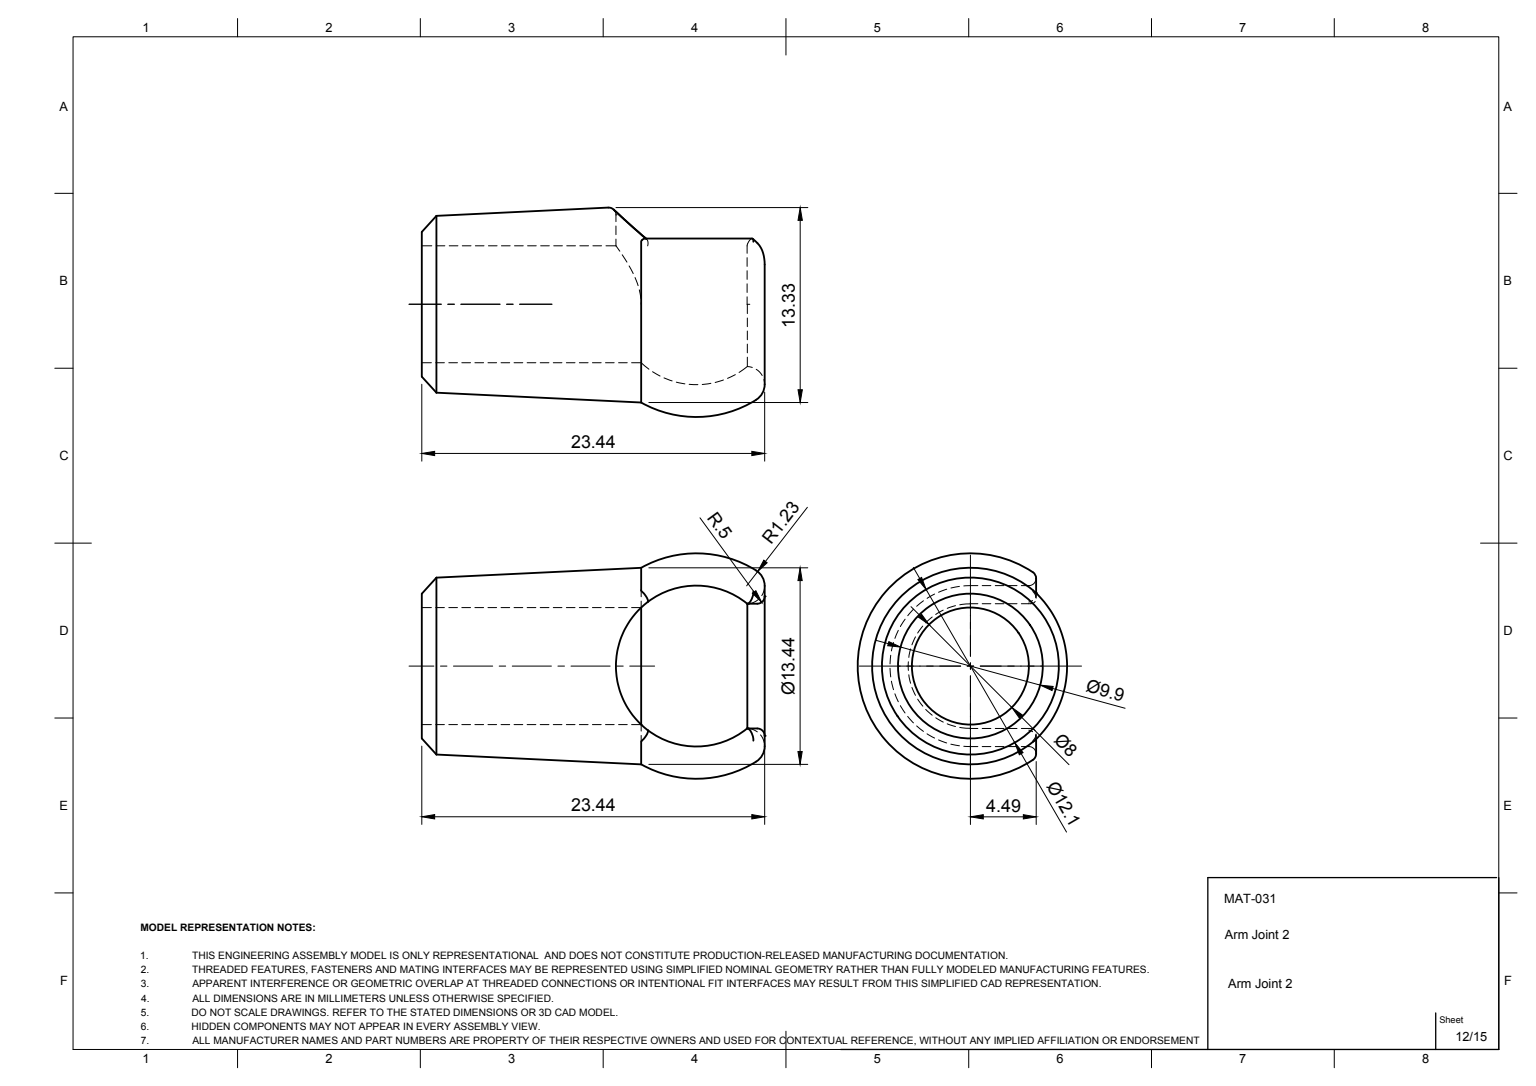
ISO-10303-21;
HEADER;
/* Generated by software containing ST-Developer
 * from STEP Tools, Inc. (www.steptools.com) 
 */

FILE_DESCRIPTION(
/* description */ ('STEP AP214'),
/* implementation_level */ '2;1');

FILE_NAME(
/* name */ 'Arm Joint 2.step',
/* time_stamp */ '2026-11-14T06:58:01-08:00',
/* author */ (''),
/* organization */ (''),
/* preprocessor_version */ 'ST-DEVELOPER v20.2',
/* originating_system */ 'Autodesk Translation Framework v15.17.0.0',
/* authorisation */ '');

FILE_SCHEMA (('AUTOMOTIVE_DESIGN { 1 0 10303 214 3 1 1 }'));
ENDSEC;

DATA;
#10=MECHANICAL_DESIGN_GEOMETRIC_PRESENTATION_REPRESENTATION('',(#1155),#38635);
#89=SPHERICAL_SURFACE('',#18166,5.5);
#90=SPHERICAL_SURFACE('',#18175,7.70789157434132);
#135=(
BOUNDED_SURFACE()
B_SPLINE_SURFACE(3,2,((#32683,#32684,#32685),(#32686,#32687,#32688),(#32689,
#32690,#32691),(#32692,#32693,#32694),(#32695,#32696,#32697),(#32698,#32699,
#32700),(#32701,#32702,#32703),(#32704,#32705,#32706),(#32707,#32708,#32709),
(#32710,#32711,#32712),(#32713,#32714,#32715),(#32716,#32717,#32718),(#32719,
#32720,#32721),(#32722,#32723,#32724),(#32725,#32726,#32727),(#32728,#32729,
#32730),(#32731,#32732,#32733),(#32734,#32735,#32736),(#32737,#32738,#32739),
(#32740,#32741,#32742),(#32743,#32744,#32745),(#32746,#32747,#32748)),
 .UNSPECIFIED.,.F.,.F.,.F.)
B_SPLINE_SURFACE_WITH_KNOTS((4,2,2,2,2,2,2,2,2,2,4),(3,3),(0.00881272913566369,
0.00928844068390005,0.00953838644963798,0.00978833221537591,0.0100382779811138,
0.0105381695125897,0.0110380610440656,0.0120378441070173,0.0125377356384932,
0.0127876814042311,0.01326339295247),(-0.00102566064560791,1.),
 .UNSPECIFIED.)
GEOMETRIC_REPRESENTATION_ITEM()
RATIONAL_B_SPLINE_SURFACE(((1.00132329066919,0.354908139032077,1.),(1.00124812393843,
0.391551219315617,1.),(1.00115915858371,0.434921000104149,1.),(1.00102358876472,
0.501010022609669,1.),(1.00097653790903,0.523946875988812,1.),(1.00088693501083,
0.567627453274935,1.),(1.00084389129738,0.588610862181495,1.),(1.00076096626522,
0.629036042047148,1.),(1.00072089412048,0.648570838919578,1.),(1.00060683104295,
0.704175525527758,1.),(1.00053863758583,0.737419199938388,1.),(1.00041471240488,
0.797831569997033,1.),(1.00035895931741,0.825010680216488,1.),(1.00021007792585,
0.897588970214807,1.),(1.00013587466058,0.933762370057051,1.),(1.00006032673641,
0.970591278572527,1.),(1.00004117816685,0.979926027666627,1.),(1.00002165568508,
0.989443055473061,1.),(1.00001667885161,0.991869215376876,1.),(1.00000682799133,
0.99667141789903,1.),(1.00000607453102,0.997038722775045,1.),(1.00001271218793,
0.993802926931325,1.)))
REPRESENTATION_ITEM('')
SURFACE()
);
#136=(
BOUNDED_SURFACE()
B_SPLINE_SURFACE(3,2,((#32822,#32823,#32824),(#32825,#32826,#32827),(#32828,
#32829,#32830),(#32831,#32832,#32833),(#32834,#32835,#32836),(#32837,#32838,
#32839),(#32840,#32841,#32842),(#32843,#32844,#32845),(#32846,#32847,#32848),
(#32849,#32850,#32851),(#32852,#32853,#32854),(#32855,#32856,#32857),(#32858,
#32859,#32860),(#32861,#32862,#32863),(#32864,#32865,#32866),(#32867,#32868,
#32869),(#32870,#32871,#32872),(#32873,#32874,#32875),(#32876,#32877,#32878),
(#32879,#32880,#32881),(#32882,#32883,#32884),(#32885,#32886,#32887),(#32888,
#32889,#32890),(#32891,#32892,#32893),(#32894,#32895,#32896),(#32897,#32898,
#32899),(#32900,#32901,#32902),(#32903,#32904,#32905)),.UNSPECIFIED.,.F.,
 .F.,.F.)
B_SPLINE_SURFACE_WITH_KNOTS((4,2,2,2,2,2,2,2,2,2,2,2,2,4),(3,3),(0.0120978781599544,
0.013608206651586,0.0151185351432177,0.0158736993890335,0.0166288636348494,
0.0173840278806652,0.018139192126481,0.0188943563722969,0.0196495206181127,
0.0204046848639285,0.0211598491097444,0.0219150133555602,0.022670177601376,
0.0241805060930077),(0.,1.00005676629322),.UNSPECIFIED.)
GEOMETRIC_REPRESENTATION_ITEM()
RATIONAL_B_SPLINE_SURFACE(((1.,0.419714375858336,1.00006588132778),(1.,
0.455258548961405,1.00006184590587),(1.,0.490259453324333,1.00005787216267),
(1.,0.554227398223351,1.00005060971644),(1.,0.583234396585999,1.00004731647689),
(1.,0.620852932125695,1.00004304554726),(1.,0.632335513594305,1.00004174190008),
(1.,0.652343207191375,1.00003947037488),(1.,0.660962788243787,1.00003849177155),
(1.,0.67512712292899,1.000036883658),(1.,0.680682058163542,1.00003625299183),
(1.,0.688032273240624,1.0000354185029),(1.,0.689900381447712,1.00003520641175),
(1.,0.689947597716664,1.00003520105116),(1.,0.688072411855674,1.00003541394586),
(1.,0.680752669873931,1.0000362449751),(1.,0.675339625853613,1.00003685953199),
(1.,0.661242565913974,1.00003846000767),(1.,0.652474855221301,1.00003945542854),
(1.,0.632370855573539,1.00004173788762),(1.,0.621020695612542,1.00004302650063),
(1.,0.596023875522447,1.00004586445427),(1.,0.582284387510476,1.00004742433388),
(1.,0.553320360279571,1.00005071269481),(1.,0.538073094759082,1.0000524437563),
(1.,0.490378194191559,1.00005785868172),(1.,0.455940368475232,1.00006176849714),
(1.,0.419656970284633,1.00006588784518)))
REPRESENTATION_ITEM('')
SURFACE()
);
#137=(
BOUNDED_SURFACE()
B_SPLINE_SURFACE(3,2,((#32908,#32909,#32910),(#32911,#32912,#32913),(#32914,
#32915,#32916),(#32917,#32918,#32919),(#32920,#32921,#32922),(#32923,#32924,
#32925),(#32926,#32927,#32928),(#32929,#32930,#32931),(#32932,#32933,#32934),
(#32935,#32936,#32937),(#32938,#32939,#32940),(#32941,#32942,#32943),(#32944,
#32945,#32946),(#32947,#32948,#32949),(#32950,#32951,#32952),(#32953,#32954,
#32955),(#32956,#32957,#32958),(#32959,#32960,#32961),(#32962,#32963,#32964),
(#32965,#32966,#32967),(#32968,#32969,#32970),(#32971,#32972,#32973)),
 .UNSPECIFIED.,.F.,.F.,.F.)
B_SPLINE_SURFACE_WITH_KNOTS((4,2,2,2,2,2,2,2,2,2,4),(3,3),(0.0086385816929815,
0.00928844068390017,0.00953838644963812,0.00978833221537607,0.010038277981114,
0.0105381695125899,0.0110380610440658,0.0120378441070176,0.0125377356384935,
0.0127876814042315,0.0134375403951501),(0.,1.00153795011474),
 .UNSPECIFIED.)
GEOMETRIC_REPRESENTATION_ITEM()
RATIONAL_B_SPLINE_SURFACE(((1.,0.317352891590616,1.0020997543974),(1.,0.359464191769642,
1.00197022423952),(1.,0.418763269709159,1.00178782619208),(1.,0.50075465721736,
1.00153562886443),(1.,0.523703248865329,1.00146504128611),(1.,0.567406180323521,
1.00133061542921),(1.,0.588400327795338,1.00126603952618),(1.,0.628846195835825,
1.0011416320714),(1.,0.648390989925248,1.00108151423477),(1.,0.704024133042094,
1.00091039223709),(1.,0.737284820387534,1.00080808568126),(1.,0.797728107356911,
1.000622168161),(1.,0.82492112688211,1.000538525146),(1.,0.897536559877894,
1.00031516731898),(1.,0.933728471984707,1.00020384460823),(1.,0.970576228230773,
1.00009050458634),(1.,0.97991575451876,1.00006177713528),(1.,0.98943765280286,
1.00003248872617),(1.,0.991865054329365,1.00002502228126),(1.,0.997822764595849,
1.00000669695888),(1.,0.996933411986155,1.00000943251877),(1.,0.988754588874827,
1.00003458976266)))
REPRESENTATION_ITEM('')
SURFACE()
);
#149=TOROIDAL_SURFACE('',#18150,6.,0.5);
#150=TOROIDAL_SURFACE('',#18161,5.48772230081581,1.23243402184158);
#151=TOROIDAL_SURFACE('',#18192,5.40661052483917,0.5);
#152=TOROIDAL_SURFACE('',#18193,6.,0.5);
#153=TOROIDAL_SURFACE('',#18194,5.40661052483917,0.5);
#878=FACE_BOUND('',#2883,.T.);
#990=B_SPLINE_CURVE_WITH_KNOTS('',3,(#32041,#32042,#32043,#32044),
 .UNSPECIFIED.,.F.,.F.,(4,4),(-0.193908494403496,-0.18144780310173),
 .UNSPECIFIED.);
#991=B_SPLINE_CURVE_WITH_KNOTS('',3,(#32046,#32047,#32048,#32049,#32050,
#32051,#32052,#32053,#32054,#32055,#32056,#32057,#32058,#32059,#32060,#32061,
#32062,#32063,#32064,#32065),.UNSPECIFIED.,.F.,.F.,(4,2,2,2,2,2,2,2,2,4),
(-0.167340420633072,-0.166972617746829,-0.154327111962806,-0.141796925934467,
-0.120672972956733,-0.101704261798647,-0.0839904703357835,-0.0660782047629785,
-0.0468280943861894,-0.0462066260650754),.UNSPECIFIED.);
#992=B_SPLINE_CURVE_WITH_KNOTS('',3,(#32071,#32072,#32073,#32074,#32075,
#32076,#32077,#32078),.UNSPECIFIED.,.F.,.F.,(4,2,2,4),(1.05683143574813,
1.07001373433151,1.09130065438089,1.09381163587351),.UNSPECIFIED.);
#993=B_SPLINE_CURVE_WITH_KNOTS('',3,(#32079,#32080,#32081,#32082,#32083,
#32084,#32085,#32086,#32087,#32088,#32089,#32090,#32091,#32092,#32093,#32094,
#32095,#32096,#32097,#32098,#32099,#32100,#32101,#32102,#32103,#32104,#32105,
#32106,#32107,#32108,#32109,#32110,#32111,#32112,#32113,#32114,#32115,#32116,
#32117,#32118,#32119,#32120,#32121,#32122,#32123,#32124,#32125,#32126,#32127,
#32128,#32129,#32130),.UNSPECIFIED.,.F.,.F.,(4,3,3,3,3,3,3,3,3,3,3,3,3,
3,3,3,3,4),(7.57505397569876E-13,9.10844499065638E-5,0.00018215489291624,
0.000272070717647245,0.000285322832162068,0.000352224089002271,0.00041905128827239,
0.000485831935717838,0.000552669909587165,0.000570645664324136,0.000642530907423814,
0.00071447615483413,0.000786742284179075,0.000855968496486203,0.00093427998969131,
0.00101288394362129,0.00109196298802677,0.00114129132864827),
 .UNSPECIFIED.);
#994=B_SPLINE_CURVE_WITH_KNOTS('',3,(#32140,#32141,#32142,#32143,#32144,
#32145,#32146,#32147,#32148,#32149,#32150,#32151,#32152,#32153,#32154,#32155,
#32156,#32157),.UNSPECIFIED.,.F.,.F.,(4,2,2,2,2,2,2,2,4),(-2.53894889799168,
-2.37885292235818,-2.21875694672469,-2.06148431010922,-1.90421167349376,
-1.7469390368783,-1.58966640026284,-1.42957042462934,-1.26947444899584),
 .UNSPECIFIED.);
#995=B_SPLINE_CURVE_WITH_KNOTS('',3,(#32161,#32162,#32163,#32164,#32165,
#32166,#32167,#32168,#32169,#32170,#32171,#32172,#32173,#32174,#32175,#32176,
#32177,#32178,#32179,#32180,#32181,#32182,#32183,#32184,#32185,#32186,#32187,
#32188,#32189,#32190,#32191,#32192,#32193,#32194,#32195,#32196,#32197,#32198,
#32199,#32200,#32201,#32202,#32203,#32204,#32205,#32206,#32207,#32208,#32209,
#32210,#32211,#32212,#32213,#32214,#32215,#32216,#32217,#32218,#32219,#32220,
#32221,#32222,#32223,#32224,#32225,#32226,#32227,#32228,#32229,#32230,#32231,
#32232,#32233,#32234,#32235,#32236,#32237,#32238,#32239,#32240,#32241,#32242,
#32243,#32244,#32245,#32246,#32247,#32248,#32249,#32250,#32251,#32252,#32253,
#32254,#32255,#32256,#32257,#32258,#32259,#32260,#32261,#32262,#32263,#32264,
#32265,#32266,#32267,#32268,#32269,#32270,#32271,#32272),.UNSPECIFIED.,
 .F.,.F.,(4,3,3,3,3,3,3,3,3,3,3,3,3,3,3,3,3,3,3,3,3,3,3,3,3,3,3,3,3,3,3,
3,3,3,3,3,3,4),(0.,0.000912210497134922,0.00137016845949825,0.0014036790570624,
0.00208601616582784,0.0021055185855936,0.00262363140207477,0.00279879558118489,
0.0028073581141248,0.00340274023561052,0.00350809265765975,0.003509197642656,
0.00395949408831714,0.0042110371711872,0.00421371707051397,0.00491287669971841,
0.00491670671448806,0.00528745106991125,0.00561471622824961,0.00561759561603492,
0.00631655575678081,0.00631897771198343,0.00671051133784849,0.00701839528531201,
0.00702163246524702,0.00772023481384321,0.00772763176352554,0.00824912212447548,
0.00842207434237441,0.00843697494939749,0.00902569097629585,0.00963836229883114,
0.00982575339943681,0.00986588374133253,0.0102491420369702,0.0106411882385985,
0.0110265915003307,0.0112294324564992),.UNSPECIFIED.);
#996=B_SPLINE_CURVE_WITH_KNOTS('',3,(#32284,#32285,#32286,#32287,#32288,
#32289,#32290,#32291,#32292,#32293,#32294,#32295,#32296,#32297,#32298,#32299,
#32300,#32301,#32302,#32303,#32304,#32305,#32306,#32307,#32308,#32309,#32310,
#32311,#32312,#32313,#32314,#32315,#32316,#32317,#32318,#32319,#32320,#32321,
#32322,#32323,#32324,#32325,#32326,#32327,#32328,#32329,#32330,#32331,#32332,
#32333,#32334,#32335,#32336,#32337,#32338,#32339,#32340,#32341,#32342,#32343,
#32344,#32345,#32346,#32347,#32348,#32349,#32350,#32351,#32352,#32353,#32354,
#32355,#32356,#32357,#32358,#32359,#32360,#32361,#32362,#32363,#32364,#32365,
#32366,#32367,#32368,#32369,#32370,#32371,#32372,#32373,#32374,#32375,#32376,
#32377,#32378,#32379,#32380),.UNSPECIFIED.,.F.,.F.,(4,3,3,3,3,3,3,3,3,3,
3,3,3,3,3,3,3,3,3,3,3,3,3,3,3,3,3,3,3,3,3,3,4),(0.,7.62914212120981E-5,
0.000184257247324592,0.000263187484407962,0.000292223073437087,0.00039911370766475,
0.000501087875789428,0.000584446146874173,0.00074654672592793,0.000907676866873101,
0.0010680512097945,0.00116889229374834,0.00140926922086005,0.00164595258360394,
0.00175333844062251,0.00197175143406078,0.0021842196106002,0.00233778458749668,
0.00254099318951238,0.0027343383349243,0.00292223073437084,0.00312940331866394,
0.00332978793388773,0.00350667688124501,0.00365713623155684,0.00380448204900645,
0.00394780253856282,0.00409112302811918,0.00423723456483772,0.00437340206388912,
0.00450594181348204,0.004633221785658,0.00467556917499335),
 .UNSPECIFIED.);
#997=B_SPLINE_CURVE_WITH_KNOTS('',3,(#32384,#32385,#32386,#32387,#32388,
#32389,#32390,#32391,#32392,#32393,#32394,#32395,#32396,#32397,#32398,#32399,
#32400,#32401,#32402,#32403,#32404,#32405,#32406,#32407,#32408,#32409,#32410,
#32411,#32412,#32413,#32414,#32415,#32416,#32417,#32418,#32419,#32420,#32421,
#32422,#32423,#32424,#32425,#32426,#32427,#32428,#32429,#32430,#32431,#32432,
#32433,#32434,#32435,#32436,#32437,#32438,#32439,#32440,#32441,#32442,#32443,
#32444,#32445,#32446,#32447,#32448,#32449,#32450,#32451,#32452,#32453,#32454,
#32455,#32456,#32457,#32458,#32459,#32460,#32461,#32462,#32463,#32464,#32465,
#32466,#32467,#32468,#32469,#32470,#32471,#32472,#32473,#32474,#32475,#32476,
#32477,#32478,#32479,#32480),.UNSPECIFIED.,.F.,.F.,(4,3,3,3,3,3,3,3,3,3,
3,3,3,3,3,3,3,3,3,3,3,3,3,3,3,3,3,3,3,3,3,3,4),(4.42269442734662E-18,0.00011510948078521,
0.000234103391159393,0.000285007760334435,0.000398078962146353,0.000512011060315604,
0.000570015520668867,0.000740289648794204,0.000914720697216612,0.001095344951612,
0.00114003104133773,0.00133186906084365,0.00152928739270689,0.00173576910686678,
0.00194759699451027,0.00216785204681413,0.00228006208267546,0.00249734619663865,
0.00272803292848229,0.00295230300576247,0.00318619806488783,0.00342009312401319,
0.00357729117862414,0.00373483837142073,0.0038935958084681,0.00399010864468205,
0.00408881194297815,0.00419123656775307,0.00427511640501648,0.00435284689245867,
0.00445648552890479,0.0045323946741616,0.00456012416535091),
 .UNSPECIFIED.);
#998=B_SPLINE_CURVE_WITH_KNOTS('',3,(#32499,#32500,#32501,#32502,#32503,
#32504,#32505,#32506),.UNSPECIFIED.,.F.,.F.,(4,2,2,4),(0.295121403805867,
0.297363449435658,0.307232092905955,0.311601659185375),.UNSPECIFIED.);
#999=B_SPLINE_CURVE_WITH_KNOTS('',3,(#32507,#32508,#32509,#32510,#32511,
#32512,#32513,#32514,#32515,#32516,#32517,#32518,#32519,#32520,#32521,#32522,
#32523,#32524,#32525,#32526,#32527,#32528,#32529,#32530,#32531,#32532),
 .UNSPECIFIED.,.F.,.F.,(4,2,2,2,2,2,2,2,2,2,2,2,4),(-7.41073495858817E-5,
0.00150429147127286,0.0030826902921316,0.00466108911299035,0.00545028852341972,
0.00623948793384909,0.00702868734427846,0.00781788675470783,0.0086070861651372,
0.00939628557556658,0.0101854849859959,0.0109746843964253,0.0125530832172841),
 .UNSPECIFIED.);
#1000=B_SPLINE_CURVE_WITH_KNOTS('',3,(#32549,#32550,#32551,#32552,#32553,
#32554,#32555,#32556,#32557,#32558,#32559,#32560,#32561,#32562,#32563,#32564,
#32565,#32566,#32567,#32568,#32569,#32570,#32571,#32572,#32573,#32574,#32575,
#32576,#32577,#32578,#32579,#32580,#32581,#32582,#32583,#32584,#32585,#32586,
#32587,#32588,#32589,#32590,#32591,#32592,#32593,#32594,#32595,#32596,#32597,
#32598,#32599,#32600,#32601,#32602,#32603,#32604,#32605,#32606),
 .UNSPECIFIED.,.F.,.F.,(4,3,3,3,3,3,3,3,3,3,3,3,3,3,3,3,3,3,3,4),(0.,0.000229129696581083,
0.000252698653230226,0.000253168160380289,0.000505898112004886,0.000506336320760579,
0.00101229703393971,0.00101267264152115,0.00202509487854447,0.00202534528304231,
0.00253149313182082,0.0030378927219851,0.00303801792456346,0.00329109194612974,
0.00354429164391778,0.00354435424532404,0.00379749110506874,0.00379752240570433,
0.00399904195215253,0.00405069056608462),.UNSPECIFIED.);
#1001=B_SPLINE_CURVE_WITH_KNOTS('',3,(#32610,#32611,#32612,#32613),
 .UNSPECIFIED.,.F.,.F.,(4,4),(-0.181459269355133,-0.168998578053366),
 .UNSPECIFIED.);
#1002=B_SPLINE_CURVE_WITH_KNOTS('',3,(#32617,#32618,#32619,#32620,#32621,
#32622,#32623,#32624,#32625,#32626,#32627,#32628,#32629,#32630,#32631,#32632,
#32633,#32634,#32635,#32636,#32637,#32638,#32639,#32640,#32641,#32642,#32643,
#32644,#32645,#32646,#32647,#32648,#32649,#32650,#32651,#32652,#32653,#32654,
#32655,#32656,#32657,#32658,#32659,#32660,#32661,#32662,#32663,#32664,#32665,
#32666,#32667,#32668,#32669,#32670,#32671,#32672,#32673,#32674,#32675,#32676,
#32677),.UNSPECIFIED.,.F.,.F.,(4,3,3,3,3,3,3,3,3,3,3,3,3,3,3,3,3,3,3,3,
4),(0.,0.000197327121899467,0.000247927056861424,0.000247930453861229,0.000495854113722848,
0.000495860907724086,0.000743791387463213,0.000991708227445701,0.000991721815445343,
0.00148758279649238,0.00198341645489141,0.00198344363088277,0.00297512468233711,
0.00297516544633371,0.00347097879605996,0.00347103971226963,0.00371890585292139,
0.00371913308887466,0.00381981107469357,0.0039024739051475,0.00396683290978282),
 .UNSPECIFIED.);
#1003=B_SPLINE_CURVE_WITH_KNOTS('',3,(#32751,#32752,#32753,#32754,#32755,
#32756,#32757,#32758,#32759,#32760,#32761,#32762,#32763,#32764,#32765,#32766,
#32767,#32768),.UNSPECIFIED.,.F.,.F.,(4,2,2,2,2,2,2,2,4),(-0.167140599481193,
-0.166773364806454,-0.146753267101867,-0.12714061423038,-0.106552389959774,
-0.0879503536354909,-0.0702956656303136,-0.0523482687226349,-0.0461614733531646),
 .UNSPECIFIED.);
#1004=B_SPLINE_CURVE_WITH_KNOTS('',3,(#32770,#32771,#32772,#32773,#32774,
#32775,#32776,#32777,#32778,#32779,#32780,#32781,#32782,#32783,#32784,#32785,
#32786,#32787,#32788,#32789,#32790,#32791,#32792,#32793,#32794,#32795,#32796,
#32797,#32798,#32799,#32800,#32801,#32802,#32803,#32804,#32805,#32806,#32807,
#32808,#32809,#32810,#32811,#32812,#32813,#32814,#32815,#32816,#32817,#32818,
#32819,#32820,#32821),.UNSPECIFIED.,.F.,.F.,(4,3,3,3,3,3,3,3,3,3,3,3,3,
3,3,3,3,4),(0.,9.10844491467422E-5,0.000182154892159899,0.000272070716897632,
0.000285322832163043,0.000352224089003363,0.000419051288273606,0.000485831935719175,
0.000552669909588621,0.000570645664326085,0.000642530907424901,0.000714476154834331,
0.000786742284178373,0.000855968496489128,0.000934279989732564,0.00101288394370409,
0.0010919629881535,0.00114129132865217),.UNSPECIFIED.);
#1029=CONICAL_SURFACE('',#18158,4.94835215326525,0.833377149502852);
#1030=CONICAL_SURFACE('',#18172,6.72023753462643,0.0479789861054062);
#1121=SHAPE_REPRESENTATION_RELATIONSHIP('SRR','None',#38694,#1135);
#1135=ADVANCED_BREP_SHAPE_REPRESENTATION('',(#1181),#38630);
#1155=STYLED_ITEM('',(#38767),#1181);
#1181=MANIFOLD_SOLID_BREP('Body1',#17621);
#1263=PLANE('',#18182);
#1264=PLANE('',#18183);
#1265=PLANE('',#18185);
#1266=PLANE('',#18187);
#1267=PLANE('',#18189);
#1852=FACE_OUTER_BOUND('',#2874,.T.);
#1853=FACE_OUTER_BOUND('',#2875,.T.);
#1854=FACE_OUTER_BOUND('',#2876,.T.);
#1855=FACE_OUTER_BOUND('',#2877,.T.);
#1856=FACE_OUTER_BOUND('',#2878,.T.);
#1857=FACE_OUTER_BOUND('',#2879,.T.);
#1858=FACE_OUTER_BOUND('',#2880,.T.);
#1859=FACE_OUTER_BOUND('',#2881,.T.);
#1860=FACE_OUTER_BOUND('',#2882,.T.);
#1861=FACE_OUTER_BOUND('',#2884,.T.);
#1862=FACE_OUTER_BOUND('',#2885,.T.);
#1863=FACE_OUTER_BOUND('',#2886,.T.);
#1864=FACE_OUTER_BOUND('',#2887,.T.);
#1865=FACE_OUTER_BOUND('',#2888,.T.);
#1866=FACE_OUTER_BOUND('',#2889,.T.);
#1867=FACE_OUTER_BOUND('',#2890,.T.);
#1868=FACE_OUTER_BOUND('',#2891,.T.);
#1869=FACE_OUTER_BOUND('',#2892,.T.);
#1870=FACE_OUTER_BOUND('',#2893,.T.);
#2874=EDGE_LOOP('',(#11893,#11894,#11895,#11896,#11897,#11898,#11899));
#2875=EDGE_LOOP('',(#11900,#11901,#11902,#11903,#11904,#11905,#11906,#11907));
#2876=EDGE_LOOP('',(#11908,#11909,#11910,#11911));
#2877=EDGE_LOOP('',(#11912,#11913,#11914,#11915,#11916,#11917));
#2878=EDGE_LOOP('',(#11918,#11919,#11920,#11921,#11922,#11923));
#2879=EDGE_LOOP('',(#11924,#11925,#11926,#11927,#11928));
#2880=EDGE_LOOP('',(#11929,#11930,#11931,#11932,#11933,#11934,#11935,#11936));
#2881=EDGE_LOOP('',(#11937,#11938,#11939,#11940,#11941,#11942,#11943,#11944,
#11945,#11946,#11947,#11948,#11949));
#2882=EDGE_LOOP('',(#11950));
#2883=EDGE_LOOP('',(#11951));
#2884=EDGE_LOOP('',(#11952,#11953,#11954,#11955,#11956));
#2885=EDGE_LOOP('',(#11957,#11958,#11959,#11960,#11961));
#2886=EDGE_LOOP('',(#11962,#11963,#11964,#11965));
#2887=EDGE_LOOP('',(#11966,#11967,#11968,#11969));
#2888=EDGE_LOOP('',(#11970,#11971,#11972,#11973));
#2889=EDGE_LOOP('',(#11974,#11975,#11976,#11977));
#2890=EDGE_LOOP('',(#11978,#11979,#11980,#11981,#11982,#11983,#11984));
#2891=EDGE_LOOP('',(#11985,#11986,#11987,#11988));
#2892=EDGE_LOOP('',(#11989,#11990,#11991,#11992));
#2893=EDGE_LOOP('',(#11993,#11994,#11995,#11996));
#3901=LINE('',#32136,#4845);
#3902=LINE('',#32160,#4846);
#3903=LINE('',#32277,#4847);
#3904=LINE('',#32490,#4848);
#3905=LINE('',#32495,#4849);
#3906=LINE('',#32547,#4850);
#3907=LINE('',#32678,#4851);
#4845=VECTOR('',#20684,1000.);
#4846=VECTOR('',#20689,1000.);
#4847=VECTOR('',#20694,4.94835215326525);
#4848=VECTOR('',#20717,4.);
#4849=VECTOR('',#20724,6.72023753462643);
#4850=VECTOR('',#20745,1000.);
#4851=VECTOR('',#20752,1000.);
#5739=CIRCLE('',#18151,5.5);
#5740=CIRCLE('',#18152,6.41621047834285);
#5741=CIRCLE('',#18153,6.41621047834285);
#5742=CIRCLE('',#18155,5.5);
#5743=CIRCLE('',#18156,5.5);
#5744=CIRCLE('',#18157,5.5);
#5745=CIRCLE('',#18159,6.04796058042142);
#5746=CIRCLE('',#18160,4.94835215326525);
#5747=CIRCLE('',#18162,1.23243402184158);
#5748=CIRCLE('',#18163,6.53216674526026);
#5749=CIRCLE('',#18164,1.23243402184158);
#5750=CIRCLE('',#18165,4.25614904904292);
#5751=CIRCLE('',#18167,5.5);
#5752=CIRCLE('',#18168,4.);
#5753=CIRCLE('',#18169,5.5);
#5754=CIRCLE('',#18171,4.);
#5755=CIRCLE('',#18173,6.72023753462643);
#5756=CIRCLE('',#18174,6.72023753462643);
#5757=CIRCLE('',#18176,5.7816585169653);
#5758=CIRCLE('',#18177,6.41621047834285);
#5759=CIRCLE('',#18178,7.70789157434132);
#5760=CIRCLE('',#18179,6.41621047834285);
#5761=CIRCLE('',#18180,7.70789157434132);
#5762=CIRCLE('',#18181,5.7816585169653);
#5763=CIRCLE('',#18184,5.40661052483917);
#5764=CIRCLE('',#18186,5.40661052483917);
#5765=CIRCLE('',#18188,0.5);
#5766=CIRCLE('',#18190,0.5);
#5767=CIRCLE('',#18191,0.5);
#5768=CIRCLE('',#18195,0.5);
#6829=VERTEX_POINT('',#32037);
#6830=VERTEX_POINT('',#32038);
#6831=VERTEX_POINT('',#32040);
#6832=VERTEX_POINT('',#32045);
#6833=VERTEX_POINT('',#32066);
#6834=VERTEX_POINT('',#32068);
#6835=VERTEX_POINT('',#32070);
#6836=VERTEX_POINT('',#32132);
#6837=VERTEX_POINT('',#32133);
#6838=VERTEX_POINT('',#32135);
#6839=VERTEX_POINT('',#32137);
#6840=VERTEX_POINT('',#32139);
#6841=VERTEX_POINT('',#32158);
#6842=VERTEX_POINT('',#32274);
#6843=VERTEX_POINT('',#32276);
#6844=VERTEX_POINT('',#32280);
#6845=VERTEX_POINT('',#32281);
#6846=VERTEX_POINT('',#32283);
#6847=VERTEX_POINT('',#32381);
#6848=VERTEX_POINT('',#32383);
#6849=VERTEX_POINT('',#32481);
#6850=VERTEX_POINT('',#32489);
#6851=VERTEX_POINT('',#32493);
#6852=VERTEX_POINT('',#32496);
#6853=VERTEX_POINT('',#32498);
#6854=VERTEX_POINT('',#32534);
#6855=VERTEX_POINT('',#32536);
#6856=VERTEX_POINT('',#32538);
#6857=VERTEX_POINT('',#32541);
#6858=VERTEX_POINT('',#32546);
#6859=VERTEX_POINT('',#32548);
#6860=VERTEX_POINT('',#32609);
#6861=VERTEX_POINT('',#32614);
#6862=VERTEX_POINT('',#32616);
#8733=EDGE_CURVE('',#6829,#6830,#5739,.T.);
#8734=EDGE_CURVE('',#6831,#6829,#990,.T.);
#8735=EDGE_CURVE('',#6832,#6831,#991,.T.);
#8736=EDGE_CURVE('',#6833,#6832,#5740,.T.);
#8737=EDGE_CURVE('',#6834,#6833,#5741,.T.);
#8738=EDGE_CURVE('',#6835,#6834,#992,.T.);
#8739=EDGE_CURVE('',#6835,#6830,#993,.T.);
#8740=EDGE_CURVE('',#6836,#6837,#5742,.T.);
#8741=EDGE_CURVE('',#6837,#6838,#3901,.T.);
#8742=EDGE_CURVE('',#6838,#6839,#5743,.T.);
#8743=EDGE_CURVE('',#6840,#6839,#994,.T.);
#8744=EDGE_CURVE('',#6840,#6841,#5744,.T.);
#8745=EDGE_CURVE('',#6829,#6841,#3902,.T.);
#8746=EDGE_CURVE('',#6830,#6836,#995,.T.);
#8747=EDGE_CURVE('',#6842,#6842,#5745,.T.);
#8748=EDGE_CURVE('',#6842,#6843,#3903,.T.);
#8749=EDGE_CURVE('',#6843,#6843,#5746,.T.);
#8750=EDGE_CURVE('',#6844,#6845,#5747,.T.);
#8751=EDGE_CURVE('',#6845,#6846,#996,.T.);
#8752=EDGE_CURVE('',#6847,#6846,#5748,.T.);
#8753=EDGE_CURVE('',#6847,#6848,#997,.T.);
#8754=EDGE_CURVE('',#6848,#6849,#5749,.T.);
#8755=EDGE_CURVE('',#6849,#6844,#5750,.T.);
#8756=EDGE_CURVE('',#6849,#6841,#5751,.T.);
#8757=EDGE_CURVE('',#6840,#6839,#5752,.T.);
#8758=EDGE_CURVE('',#6838,#6844,#5753,.T.);
#8759=EDGE_CURVE('',#6839,#6850,#3904,.T.);
#8760=EDGE_CURVE('',#6850,#6850,#5754,.T.);
#8761=EDGE_CURVE('',#6834,#6851,#5755,.T.);
#8762=EDGE_CURVE('',#6851,#6842,#3905,.T.);
#8763=EDGE_CURVE('',#6851,#6852,#5756,.T.);
#8764=EDGE_CURVE('',#6852,#6853,#998,.T.);
#8765=EDGE_CURVE('',#6853,#6835,#999,.T.);
#8766=EDGE_CURVE('',#6846,#6854,#5757,.T.);
#8767=EDGE_CURVE('',#6854,#6855,#5758,.T.);
#8768=EDGE_CURVE('',#6856,#6855,#5759,.T.);
#8769=EDGE_CURVE('',#6855,#6852,#5760,.T.);
#8770=EDGE_CURVE('',#6833,#6857,#5761,.T.);
#8771=EDGE_CURVE('',#6832,#6847,#5762,.T.);
#8772=EDGE_CURVE('',#6841,#6858,#3906,.T.);
#8773=EDGE_CURVE('',#6858,#6859,#1000,.T.);
#8774=EDGE_CURVE('',#6859,#6831,#5763,.T.);
#8775=EDGE_CURVE('',#6837,#6860,#1001,.T.);
#8776=EDGE_CURVE('',#6860,#6861,#5764,.T.);
#8777=EDGE_CURVE('',#6861,#6862,#1002,.T.);
#8778=EDGE_CURVE('',#6862,#6838,#3907,.T.);
#8779=EDGE_CURVE('',#6862,#6845,#5765,.T.);
#8780=EDGE_CURVE('',#6848,#6858,#5766,.T.);
#8781=EDGE_CURVE('',#6846,#6861,#5767,.T.);
#8782=EDGE_CURVE('',#6854,#6860,#1003,.T.);
#8783=EDGE_CURVE('',#6853,#6836,#1004,.T.);
#8784=EDGE_CURVE('',#6847,#6859,#5768,.T.);
#11893=ORIENTED_EDGE('',*,*,#8733,.F.);
#11894=ORIENTED_EDGE('',*,*,#8734,.F.);
#11895=ORIENTED_EDGE('',*,*,#8735,.F.);
#11896=ORIENTED_EDGE('',*,*,#8736,.F.);
#11897=ORIENTED_EDGE('',*,*,#8737,.F.);
#11898=ORIENTED_EDGE('',*,*,#8738,.F.);
#11899=ORIENTED_EDGE('',*,*,#8739,.T.);
#11900=ORIENTED_EDGE('',*,*,#8740,.T.);
#11901=ORIENTED_EDGE('',*,*,#8741,.T.);
#11902=ORIENTED_EDGE('',*,*,#8742,.T.);
#11903=ORIENTED_EDGE('',*,*,#8743,.F.);
#11904=ORIENTED_EDGE('',*,*,#8744,.T.);
#11905=ORIENTED_EDGE('',*,*,#8745,.F.);
#11906=ORIENTED_EDGE('',*,*,#8733,.T.);
#11907=ORIENTED_EDGE('',*,*,#8746,.T.);
#11908=ORIENTED_EDGE('',*,*,#8747,.F.);
#11909=ORIENTED_EDGE('',*,*,#8748,.T.);
#11910=ORIENTED_EDGE('',*,*,#8749,.F.);
#11911=ORIENTED_EDGE('',*,*,#8748,.F.);
#11912=ORIENTED_EDGE('',*,*,#8750,.T.);
#11913=ORIENTED_EDGE('',*,*,#8751,.T.);
#11914=ORIENTED_EDGE('',*,*,#8752,.F.);
#11915=ORIENTED_EDGE('',*,*,#8753,.T.);
#11916=ORIENTED_EDGE('',*,*,#8754,.T.);
#11917=ORIENTED_EDGE('',*,*,#8755,.T.);
#11918=ORIENTED_EDGE('',*,*,#8755,.F.);
#11919=ORIENTED_EDGE('',*,*,#8756,.T.);
#11920=ORIENTED_EDGE('',*,*,#8744,.F.);
#11921=ORIENTED_EDGE('',*,*,#8757,.T.);
#11922=ORIENTED_EDGE('',*,*,#8742,.F.);
#11923=ORIENTED_EDGE('',*,*,#8758,.T.);
#11924=ORIENTED_EDGE('',*,*,#8743,.T.);
#11925=ORIENTED_EDGE('',*,*,#8759,.T.);
#11926=ORIENTED_EDGE('',*,*,#8760,.T.);
#11927=ORIENTED_EDGE('',*,*,#8759,.F.);
#11928=ORIENTED_EDGE('',*,*,#8757,.F.);
#11929=ORIENTED_EDGE('',*,*,#8761,.T.);
#11930=ORIENTED_EDGE('',*,*,#8762,.T.);
#11931=ORIENTED_EDGE('',*,*,#8747,.T.);
#11932=ORIENTED_EDGE('',*,*,#8762,.F.);
#11933=ORIENTED_EDGE('',*,*,#8763,.T.);
#11934=ORIENTED_EDGE('',*,*,#8764,.T.);
#11935=ORIENTED_EDGE('',*,*,#8765,.T.);
#11936=ORIENTED_EDGE('',*,*,#8738,.T.);
#11937=ORIENTED_EDGE('',*,*,#8752,.T.);
#11938=ORIENTED_EDGE('',*,*,#8766,.T.);
#11939=ORIENTED_EDGE('',*,*,#8767,.T.);
#11940=ORIENTED_EDGE('',*,*,#8768,.F.);
#11941=ORIENTED_EDGE('',*,*,#8768,.T.);
#11942=ORIENTED_EDGE('',*,*,#8769,.T.);
#11943=ORIENTED_EDGE('',*,*,#8763,.F.);
#11944=ORIENTED_EDGE('',*,*,#8761,.F.);
#11945=ORIENTED_EDGE('',*,*,#8737,.T.);
#11946=ORIENTED_EDGE('',*,*,#8770,.T.);
#11947=ORIENTED_EDGE('',*,*,#8770,.F.);
#11948=ORIENTED_EDGE('',*,*,#8736,.T.);
#11949=ORIENTED_EDGE('',*,*,#8771,.T.);
#11950=ORIENTED_EDGE('',*,*,#8749,.T.);
#11951=ORIENTED_EDGE('',*,*,#8760,.F.);
#11952=ORIENTED_EDGE('',*,*,#8772,.T.);
#11953=ORIENTED_EDGE('',*,*,#8773,.T.);
#11954=ORIENTED_EDGE('',*,*,#8774,.T.);
#11955=ORIENTED_EDGE('',*,*,#8734,.T.);
#11956=ORIENTED_EDGE('',*,*,#8745,.T.);
#11957=ORIENTED_EDGE('',*,*,#8741,.F.);
#11958=ORIENTED_EDGE('',*,*,#8775,.T.);
#11959=ORIENTED_EDGE('',*,*,#8776,.T.);
#11960=ORIENTED_EDGE('',*,*,#8777,.T.);
#11961=ORIENTED_EDGE('',*,*,#8778,.T.);
#11962=ORIENTED_EDGE('',*,*,#8778,.F.);
#11963=ORIENTED_EDGE('',*,*,#8779,.T.);
#11964=ORIENTED_EDGE('',*,*,#8750,.F.);
#11965=ORIENTED_EDGE('',*,*,#8758,.F.);
#11966=ORIENTED_EDGE('',*,*,#8754,.F.);
#11967=ORIENTED_EDGE('',*,*,#8780,.T.);
#11968=ORIENTED_EDGE('',*,*,#8772,.F.);
#11969=ORIENTED_EDGE('',*,*,#8756,.F.);
#11970=ORIENTED_EDGE('',*,*,#8779,.F.);
#11971=ORIENTED_EDGE('',*,*,#8777,.F.);
#11972=ORIENTED_EDGE('',*,*,#8781,.F.);
#11973=ORIENTED_EDGE('',*,*,#8751,.F.);
#11974=ORIENTED_EDGE('',*,*,#8781,.T.);
#11975=ORIENTED_EDGE('',*,*,#8776,.F.);
#11976=ORIENTED_EDGE('',*,*,#8782,.F.);
#11977=ORIENTED_EDGE('',*,*,#8766,.F.);
#11978=ORIENTED_EDGE('',*,*,#8775,.F.);
#11979=ORIENTED_EDGE('',*,*,#8740,.F.);
#11980=ORIENTED_EDGE('',*,*,#8783,.F.);
#11981=ORIENTED_EDGE('',*,*,#8764,.F.);
#11982=ORIENTED_EDGE('',*,*,#8769,.F.);
#11983=ORIENTED_EDGE('',*,*,#8767,.F.);
#11984=ORIENTED_EDGE('',*,*,#8782,.T.);
#11985=ORIENTED_EDGE('',*,*,#8783,.T.);
#11986=ORIENTED_EDGE('',*,*,#8746,.F.);
#11987=ORIENTED_EDGE('',*,*,#8739,.F.);
#11988=ORIENTED_EDGE('',*,*,#8765,.F.);
#11989=ORIENTED_EDGE('',*,*,#8735,.T.);
#11990=ORIENTED_EDGE('',*,*,#8774,.F.);
#11991=ORIENTED_EDGE('',*,*,#8784,.F.);
#11992=ORIENTED_EDGE('',*,*,#8771,.F.);
#11993=ORIENTED_EDGE('',*,*,#8784,.T.);
#11994=ORIENTED_EDGE('',*,*,#8773,.F.);
#11995=ORIENTED_EDGE('',*,*,#8780,.F.);
#11996=ORIENTED_EDGE('',*,*,#8753,.F.);
#16341=CYLINDRICAL_SURFACE('',#18154,5.5);
#16342=CYLINDRICAL_SURFACE('',#18170,4.);
#16811=ADVANCED_FACE('',(#1852),#149,.T.);
#16812=ADVANCED_FACE('',(#1853),#16341,.F.);
#16813=ADVANCED_FACE('',(#1854),#1029,.T.);
#16814=ADVANCED_FACE('',(#1855),#150,.T.);
#16815=ADVANCED_FACE('',(#1856),#89,.F.);
#16816=ADVANCED_FACE('',(#1857),#16342,.F.);
#16817=ADVANCED_FACE('',(#1858),#1030,.T.);
#16818=ADVANCED_FACE('',(#1859),#90,.T.);
#16819=ADVANCED_FACE('',(#1860,#878),#1263,.F.);
#16820=ADVANCED_FACE('',(#1861),#1264,.F.);
#16821=ADVANCED_FACE('',(#1862),#1265,.F.);
#16822=ADVANCED_FACE('',(#1863),#1266,.F.);
#16823=ADVANCED_FACE('',(#1864),#1267,.F.);
#16824=ADVANCED_FACE('',(#1865),#135,.T.);
#16825=ADVANCED_FACE('',(#1866),#151,.T.);
#16826=ADVANCED_FACE('',(#1867),#152,.T.);
#16827=ADVANCED_FACE('',(#1868),#136,.T.);
#16828=ADVANCED_FACE('',(#1869),#153,.T.);
#16829=ADVANCED_FACE('',(#1870),#137,.T.);
#17621=CLOSED_SHELL('',(#16811,#16812,#16813,#16814,#16815,#16816,#16817,
#16818,#16819,#16820,#16821,#16822,#16823,#16824,#16825,#16826,#16827,#16828,
#16829));
#18149=AXIS2_PLACEMENT_3D('',#32035,#20670,#20671);
#18150=AXIS2_PLACEMENT_3D('',#32036,#20672,#20673);
#18151=AXIS2_PLACEMENT_3D('',#32039,#20674,#20675);
#18152=AXIS2_PLACEMENT_3D('',#32067,#20676,#20677);
#18153=AXIS2_PLACEMENT_3D('',#32069,#20678,#20679);
#18154=AXIS2_PLACEMENT_3D('',#32131,#20680,#20681);
#18155=AXIS2_PLACEMENT_3D('',#32134,#20682,#20683);
#18156=AXIS2_PLACEMENT_3D('',#32138,#20685,#20686);
#18157=AXIS2_PLACEMENT_3D('',#32159,#20687,#20688);
#18158=AXIS2_PLACEMENT_3D('',#32273,#20690,#20691);
#18159=AXIS2_PLACEMENT_3D('',#32275,#20692,#20693);
#18160=AXIS2_PLACEMENT_3D('',#32278,#20695,#20696);
#18161=AXIS2_PLACEMENT_3D('',#32279,#20697,#20698);
#18162=AXIS2_PLACEMENT_3D('',#32282,#20699,#20700);
#18163=AXIS2_PLACEMENT_3D('',#32382,#20701,#20702);
#18164=AXIS2_PLACEMENT_3D('',#32482,#20703,#20704);
#18165=AXIS2_PLACEMENT_3D('',#32483,#20705,#20706);
#18166=AXIS2_PLACEMENT_3D('',#32484,#20707,#20708);
#18167=AXIS2_PLACEMENT_3D('',#32485,#20709,#20710);
#18168=AXIS2_PLACEMENT_3D('',#32486,#20711,#20712);
#18169=AXIS2_PLACEMENT_3D('',#32487,#20713,#20714);
#18170=AXIS2_PLACEMENT_3D('',#32488,#20715,#20716);
#18171=AXIS2_PLACEMENT_3D('',#32491,#20718,#20719);
#18172=AXIS2_PLACEMENT_3D('',#32492,#20720,#20721);
#18173=AXIS2_PLACEMENT_3D('',#32494,#20722,#20723);
#18174=AXIS2_PLACEMENT_3D('',#32497,#20725,#20726);
#18175=AXIS2_PLACEMENT_3D('',#32533,#20727,#20728);
#18176=AXIS2_PLACEMENT_3D('',#32535,#20729,#20730);
#18177=AXIS2_PLACEMENT_3D('',#32537,#20731,#20732);
#18178=AXIS2_PLACEMENT_3D('',#32539,#20733,#20734);
#18179=AXIS2_PLACEMENT_3D('',#32540,#20735,#20736);
#18180=AXIS2_PLACEMENT_3D('',#32542,#20737,#20738);
#18181=AXIS2_PLACEMENT_3D('',#32543,#20739,#20740);
#18182=AXIS2_PLACEMENT_3D('',#32544,#20741,#20742);
#18183=AXIS2_PLACEMENT_3D('',#32545,#20743,#20744);
#18184=AXIS2_PLACEMENT_3D('',#32607,#20746,#20747);
#18185=AXIS2_PLACEMENT_3D('',#32608,#20748,#20749);
#18186=AXIS2_PLACEMENT_3D('',#32615,#20750,#20751);
#18187=AXIS2_PLACEMENT_3D('',#32679,#20753,#20754);
#18188=AXIS2_PLACEMENT_3D('',#32680,#20755,#20756);
#18189=AXIS2_PLACEMENT_3D('',#32681,#20757,#20758);
#18190=AXIS2_PLACEMENT_3D('',#32682,#20759,#20760);
#18191=AXIS2_PLACEMENT_3D('',#32749,#20761,#20762);
#18192=AXIS2_PLACEMENT_3D('',#32750,#20763,#20764);
#18193=AXIS2_PLACEMENT_3D('',#32769,#20765,#20766);
#18194=AXIS2_PLACEMENT_3D('',#32906,#20767,#20768);
#18195=AXIS2_PLACEMENT_3D('',#32907,#20769,#20770);
#20670=DIRECTION('axis',(0.,0.,1.));
#20671=DIRECTION('refdir',(1.,0.,0.));
#20672=DIRECTION('center_axis',(0.,1.,0.));
#20673=DIRECTION('ref_axis',(0.,0.,1.));
#20674=DIRECTION('center_axis',(0.,-1.,0.));
#20675=DIRECTION('ref_axis',(0.,0.,1.));
#20676=DIRECTION('center_axis',(0.,1.,0.));
#20677=DIRECTION('ref_axis',(0.,0.,1.));
#20678=DIRECTION('center_axis',(0.,1.,0.));
#20679=DIRECTION('ref_axis',(0.,0.,1.));
#20680=DIRECTION('center_axis',(0.,1.,0.));
#20681=DIRECTION('ref_axis',(-1.,0.,-1.83697019872103E-16));
#20682=DIRECTION('center_axis',(0.,-1.,0.));
#20683=DIRECTION('ref_axis',(1.89242561015652E-15,0.,1.));
#20684=DIRECTION('',(0.,1.,0.));
#20685=DIRECTION('center_axis',(0.,1.,0.));
#20686=DIRECTION('ref_axis',(0.,0.,1.));
#20687=DIRECTION('center_axis',(0.,1.,0.));
#20688=DIRECTION('ref_axis',(0.,0.,1.));
#20689=DIRECTION('',(0.,1.,0.));
#20690=DIRECTION('center_axis',(1.,0.,0.));
#20691=DIRECTION('ref_axis',(0.,0.,-1.));
#20692=DIRECTION('center_axis',(1.,0.,0.));
#20693=DIRECTION('ref_axis',(0.,0.,1.));
#20694=DIRECTION('',(-0.672379811723126,9.06491294391023E-17,-0.740206315014384));
#20695=DIRECTION('center_axis',(-1.,0.,0.));
#20696=DIRECTION('ref_axis',(0.,0.,-1.));
#20697=DIRECTION('center_axis',(-1.,0.,0.));
#20698=DIRECTION('ref_axis',(0.,1.,6.12323399573677E-17));
#20699=DIRECTION('center_axis',(0.,1.,0.));
#20700=DIRECTION('ref_axis',(0.,0.,1.));
#20701=DIRECTION('center_axis',(-1.,0.,0.));
#20702=DIRECTION('ref_axis',(0.,0.,1.));
#20703=DIRECTION('center_axis',(0.,1.,0.));
#20704=DIRECTION('ref_axis',(0.,0.,1.));
#20705=DIRECTION('center_axis',(-1.,0.,0.));
#20706=DIRECTION('ref_axis',(0.,0.,1.));
#20707=DIRECTION('center_axis',(1.,6.12323399573677E-17,-7.49879891330929E-33));
#20708=DIRECTION('ref_axis',(0.,1.,-1.22464679914735E-16));
#20709=DIRECTION('center_axis',(0.,-1.,0.));
#20710=DIRECTION('ref_axis',(0.,0.,1.));
#20711=DIRECTION('center_axis',(-1.,0.,0.));
#20712=DIRECTION('ref_axis',(0.,0.,1.));
#20713=DIRECTION('center_axis',(0.,-1.,0.));
#20714=DIRECTION('ref_axis',(-5.56057725117657E-13,0.,1.));
#20715=DIRECTION('center_axis',(-1.,0.,0.));
#20716=DIRECTION('ref_axis',(0.,0.,1.));
#20717=DIRECTION('',(-1.,0.,0.));
#20718=DIRECTION('center_axis',(-1.,0.,0.));
#20719=DIRECTION('ref_axis',(0.,0.,1.));
#20720=DIRECTION('center_axis',(1.,0.,0.));
#20721=DIRECTION('ref_axis',(0.,0.,-1.));
#20722=DIRECTION('center_axis',(-1.,0.,0.));
#20723=DIRECTION('ref_axis',(0.,0.,1.));
#20724=DIRECTION('',(-0.998849229226133,5.87347712983446E-18,-0.0479605804214227));
#20725=DIRECTION('center_axis',(-1.,0.,0.));
#20726=DIRECTION('ref_axis',(0.,0.,1.));
#20727=DIRECTION('center_axis',(0.,6.12323399573676E-17,-1.));
#20728=DIRECTION('ref_axis',(0.,1.,0.));
#20729=DIRECTION('center_axis',(0.,0.,-1.));
#20730=DIRECTION('ref_axis',(1.,0.,0.));
#20731=DIRECTION('center_axis',(0.,1.,0.));
#20732=DIRECTION('ref_axis',(0.,0.,1.));
#20733=DIRECTION('center_axis',(-1.,0.,0.));
#20734=DIRECTION('ref_axis',(0.,-1.,0.));
#20735=DIRECTION('center_axis',(0.,1.,0.));
#20736=DIRECTION('ref_axis',(0.,0.,1.));
#20737=DIRECTION('center_axis',(-1.,0.,0.));
#20738=DIRECTION('ref_axis',(0.,-1.,0.));
#20739=DIRECTION('center_axis',(0.,0.,1.));
#20740=DIRECTION('ref_axis',(-1.,0.,0.));
#20741=DIRECTION('center_axis',(1.,0.,0.));
#20742=DIRECTION('ref_axis',(0.,0.,-1.));
#20743=DIRECTION('center_axis',(0.,0.,1.));
#20744=DIRECTION('ref_axis',(1.,0.,0.));
#20745=DIRECTION('',(1.,0.,0.));
#20746=DIRECTION('center_axis',(0.,0.,-1.));
#20747=DIRECTION('ref_axis',(1.,8.88178419700125E-16,0.));
#20748=DIRECTION('center_axis',(0.,0.,-1.));
#20749=DIRECTION('ref_axis',(-1.,0.,0.));
#20750=DIRECTION('center_axis',(0.,0.,1.));
#20751=DIRECTION('ref_axis',(-1.,-1.24344978758018E-14,0.));
#20752=DIRECTION('',(-1.,0.,0.));
#20753=DIRECTION('center_axis',(0.,1.,0.));
#20754=DIRECTION('ref_axis',(0.,0.,1.));
#20755=DIRECTION('center_axis',(0.,1.,0.));
#20756=DIRECTION('ref_axis',(0.,0.,1.));
#20757=DIRECTION('center_axis',(0.,1.,0.));
#20758=DIRECTION('ref_axis',(0.,0.,1.));
#20759=DIRECTION('center_axis',(0.,1.,0.));
#20760=DIRECTION('ref_axis',(0.,0.,1.));
#20761=DIRECTION('center_axis',(-0.706501481417622,-0.707711563247843,-1.83312916504447E-15));
#20762=DIRECTION('ref_axis',(0.707711563247843,-0.706501481417622,-1.95764081482192E-30));
#20763=DIRECTION('center_axis',(0.,0.,-1.));
#20764=DIRECTION('ref_axis',(-1.,0.,0.));
#20765=DIRECTION('center_axis',(0.,1.,0.));
#20766=DIRECTION('ref_axis',(0.0232101926599813,0.,-0.999730607192101));
#20767=DIRECTION('center_axis',(0.,0.,1.));
#20768=DIRECTION('ref_axis',(1.,0.,0.));
#20769=DIRECTION('center_axis',(0.706501481417621,0.707711563247844,0.));
#20770=DIRECTION('ref_axis',(-0.707711563247844,0.706501481417621,0.));
#32035=CARTESIAN_POINT('',(0.,0.,0.));
#32036=CARTESIAN_POINT('Origin',(14.8870768733179,-3.99420842564088,0.));
#32037=CARTESIAN_POINT('',(18.3575990203927,-3.99420842564088,4.26678755349543));
#32038=CARTESIAN_POINT('',(11.5587496781628,-3.99420842549338,4.37861311631065));
#32039=CARTESIAN_POINT('Origin',(14.8870768733179,-3.99420842564088,0.));
#32040=CARTESIAN_POINT('',(18.3843475112712,-4.12317055822481,4.26678755349543));
#32041=CARTESIAN_POINT('Ctrl Pts',(18.3843475112712,-4.1231705582248,4.26678755349543));
#32042=CARTESIAN_POINT('Ctrl Pts',(18.3672627745756,-4.08260100655593,4.26678755349543));
#32043=CARTESIAN_POINT('Ctrl Pts',(18.3575990203927,-4.03574406331344,4.26678755349543));
#32044=CARTESIAN_POINT('Ctrl Pts',(18.3575990203927,-3.99420842564088,4.26678755349543));
#32045=CARTESIAN_POINT('',(18.7837086993174,-4.27128032554705,5.09745204146194));
#32046=CARTESIAN_POINT('Ctrl Pts',(18.7837086993174,-4.27128032554705,5.09745204146194));
#32047=CARTESIAN_POINT('Ctrl Pts',(18.7837837490088,-4.27218840717948,5.09663376751006));
#32048=CARTESIAN_POINT('Ctrl Pts',(18.7838568749948,-4.27309451506193,5.09581312836018));
#32049=CARTESIAN_POINT('Ctrl Pts',(18.786376054168,-4.30508335769532,5.0666946999686));
#32050=CARTESIAN_POINT('Ctrl Pts',(18.7865447928184,-4.33378349175756,5.03565092415356));
#32051=CARTESIAN_POINT('Ctrl Pts',(18.7822885734857,-4.38502690350443,4.96945449120915));
#32052=CARTESIAN_POINT('Ctrl Pts',(18.7779104286292,-4.40756216172138,4.93442106198759));
#32053=CARTESIAN_POINT('Ctrl Pts',(18.7601365382803,-4.4586258081985,4.8363053847714));
#32054=CARTESIAN_POINT('Ctrl Pts',(18.7426983881329,-4.48040963095378,4.77095332236947));
#32055=CARTESIAN_POINT('Ctrl Pts',(18.6987452289246,-4.49763058563495,4.64635114121833));
#32056=CARTESIAN_POINT('Ctrl Pts',(18.6736500581964,-4.49538158540805,4.58805456925361));
#32057=CARTESIAN_POINT('Ctrl Pts',(18.6187727586818,-4.46886694818906,4.48266333773381));
#32058=CARTESIAN_POINT('Ctrl Pts',(18.5900193347752,-4.44634242811073,4.43625626352526));
#32059=CARTESIAN_POINT('Ctrl Pts',(18.5302580379935,-4.38241110798174,4.35685111603697));
#32060=CARTESIAN_POINT('Ctrl Pts',(18.500152649712,-4.34177888816883,4.32523467597912));
#32061=CARTESIAN_POINT('Ctrl Pts',(18.4403522870749,-4.24412140399772,4.27947358970446));
#32062=CARTESIAN_POINT('Ctrl Pts',(18.4118332395335,-4.18772090860718,4.26754505508647));
#32063=CARTESIAN_POINT('Ctrl Pts',(18.3859538609649,-4.12697400251701,4.26679918369438));
#32064=CARTESIAN_POINT('Ctrl Pts',(18.3851486227203,-4.12507288384488,4.26678755349543));
#32065=CARTESIAN_POINT('Ctrl Pts',(18.3843475112712,-4.1231705582248,4.26678755349543));
#32066=CARTESIAN_POINT('',(14.8870768733179,-4.27128032554705,6.41621047834285));
#32067=CARTESIAN_POINT('Origin',(14.8870768733179,-4.27128032554705,0.));
#32068=CARTESIAN_POINT('',(11.1121596556826,-4.27128032554705,5.18823254127999));
#32069=CARTESIAN_POINT('Origin',(14.8870768733179,-4.27128032554705,0.));
#32070=CARTESIAN_POINT('',(11.1585526808199,-4.38134327817891,5.09856534363104));
#32071=CARTESIAN_POINT('Ctrl Pts',(11.1585526808199,-4.3813432781789,5.09856534363105));
#32072=CARTESIAN_POINT('Ctrl Pts',(11.1473312438077,-4.36992324654723,5.10766848669372));
#32073=CARTESIAN_POINT('Ctrl Pts',(11.1380491180006,-4.35765259554692,5.11756292166355));
#32074=CARTESIAN_POINT('Ctrl Pts',(11.1191192706006,-4.32341816221833,5.14537473079008));
#32075=CARTESIAN_POINT('Ctrl Pts',(11.1134224194163,-4.30138253065776,5.163462535227));
#32076=CARTESIAN_POINT('Ctrl Pts',(11.1122215415905,-4.27651763887363,5.18392138130289));
#32077=CARTESIAN_POINT('Ctrl Pts',(11.1121596556826,-4.27389704286368,5.18607829451038));
#32078=CARTESIAN_POINT('Ctrl Pts',(11.1121596556826,-4.27128032554705,5.18823254127999));
#32079=CARTESIAN_POINT('Ctrl Pts',(11.1585526808199,-4.3813432781789,5.09856534363102));
#32080=CARTESIAN_POINT('Ctrl Pts',(11.1773095549183,-4.40043210755625,5.08334924344489));
#32081=CARTESIAN_POINT('Ctrl Pts',(11.1965634151784,-4.4173731502363,5.06638959987712));
#32082=CARTESIAN_POINT('Ctrl Pts',(11.2160327365605,-4.43193019076584,5.04794583007894));
#32083=CARTESIAN_POINT('Ctrl Pts',(11.2354990641271,-4.44648499284589,5.02950489639618));
#32084=CARTESIAN_POINT('Ctrl Pts',(11.2551808642034,-4.45865655252623,5.00958029965859));
#32085=CARTESIAN_POINT('Ctrl Pts',(11.274792429352,-4.46825273239085,4.9884587446323));
#32086=CARTESIAN_POINT('Ctrl Pts',(11.2941553532197,-4.47772724902083,4.96760497498952));
#32087=CARTESIAN_POINT('Ctrl Pts',(11.3134499546024,-4.48469120840074,4.94558444999912));
#32088=CARTESIAN_POINT('Ctrl Pts',(11.3323953871065,-4.4890027089001,4.92269940887843));
#32089=CARTESIAN_POINT('Ctrl Pts',(11.3351876324295,-4.48963815320058,4.91932653000516));
#32090=CARTESIAN_POINT('Ctrl Pts',(11.337972280205,-4.49021605981353,4.91593491859636));
#32091=CARTESIAN_POINT('Ctrl Pts',(11.3407484170913,-4.49073605743567,4.91252559036269));
#32092=CARTESIAN_POINT('Ctrl Pts',(11.3547633161211,-4.49336118525475,4.89531412244499));
#32093=CARTESIAN_POINT('Ctrl Pts',(11.3685552099561,-4.49450846568624,4.87762256908791));
#32094=CARTESIAN_POINT('Ctrl Pts',(11.3819878602125,-4.49414152262893,4.85965719763341));
#32095=CARTESIAN_POINT('Ctrl Pts',(11.395405640951,-4.49377498576595,4.84171171327548));
#32096=CARTESIAN_POINT('Ctrl Pts',(11.408464565942,-4.49189752730246,4.82349370723299));
#32097=CARTESIAN_POINT('Ctrl Pts',(11.4210277728039,-4.4885248109505,4.80521097378518));
#32098=CARTESIAN_POINT('Ctrl Pts',(11.4335822281363,-4.48515444403263,4.78694097608885));
#32099=CARTESIAN_POINT('Ctrl Pts',(11.4456412560887,-4.4802910478885,4.76860702043866));
#32100=CARTESIAN_POINT('Ctrl Pts',(11.4570732740609,-4.47400139883477,4.75040836654866));
#32101=CARTESIAN_POINT('Ctrl Pts',(11.4685151056053,-4.46770635056582,4.73219409041199));
#32102=CARTESIAN_POINT('Ctrl Pts',(11.4793284781842,-4.45998292162542,4.71411597746148));
#32103=CARTESIAN_POINT('Ctrl Pts',(11.4893922899608,-4.45094580241425,4.69635581925144));
#32104=CARTESIAN_POINT('Ctrl Pts',(11.4920989042063,-4.4485153122443,4.69157930928875));
#32105=CARTESIAN_POINT('Ctrl Pts',(11.4947513791458,-4.44599005094235,4.68682566810614));
#32106=CARTESIAN_POINT('Ctrl Pts',(11.4973475437826,-4.44337278307003,4.68209812382832));
#32107=CARTESIAN_POINT('Ctrl Pts',(11.5077296350369,-4.43290629974226,4.66319262168678));
#32108=CARTESIAN_POINT('Ctrl Pts',(11.5172734125896,-4.42090574709578,4.6446023839419));
#32109=CARTESIAN_POINT('Ctrl Pts',(11.5258955869574,-4.40751314754861,4.62655201641239));
#32110=CARTESIAN_POINT('Ctrl Pts',(11.5345249584578,-4.3941093688822,4.60848658181469));
#32111=CARTESIAN_POINT('Ctrl Pts',(11.5422308699739,-4.37931167764824,4.5909623828728));
#32112=CARTESIAN_POINT('Ctrl Pts',(11.5489433162914,-4.36330323603289,4.57417465116161));
#32113=CARTESIAN_POINT('Ctrl Pts',(11.5556857006915,-4.34722339540369,4.55731204473634));
#32114=CARTESIAN_POINT('Ctrl Pts',(11.5614254453185,-4.32992254541911,4.54119286157319));
#32115=CARTESIAN_POINT('Ctrl Pts',(11.5661098411332,-4.31161973967048,4.52597841654563));
#32116=CARTESIAN_POINT('Ctrl Pts',(11.5705971850955,-4.29408685216071,4.51140397605518));
#32117=CARTESIAN_POINT('Ctrl Pts',(11.5741160472691,-4.27563526415159,4.49765968025081));
#32118=CARTESIAN_POINT('Ctrl Pts',(11.5766390463652,-4.25647826147709,4.48485227018126));
#32119=CARTESIAN_POINT('Ctrl Pts',(11.5794931650578,-4.23480708469628,4.47036400954688));
#32120=CARTESIAN_POINT('Ctrl Pts',(11.5810960704826,-4.21214692060508,4.4570253967079));
#32121=CARTESIAN_POINT('Ctrl Pts',(11.5814513272692,-4.18878092059738,4.44498843498031));
#32122=CARTESIAN_POINT('Ctrl Pts',(11.5818079107915,-4.1653276583371,4.43290652022721));
#32123=CARTESIAN_POINT('Ctrl Pts',(11.5809072718065,-4.14116392290607,4.42213601639323));
#32124=CARTESIAN_POINT('Ctrl Pts',(11.5787776008328,-4.1165901294392,4.41278615288452));
#32125=CARTESIAN_POINT('Ctrl Pts',(11.5766350579062,-4.09186780940795,4.40337977782801));
#32126=CARTESIAN_POINT('Ctrl Pts',(11.5732483837397,-4.06673113295231,4.39541118325963));
#32127=CARTESIAN_POINT('Ctrl Pts',(11.568674438697,-4.04149025084392,4.38894711814017));
#32128=CARTESIAN_POINT('Ctrl Pts',(11.5658212792949,-4.02574536116308,4.38491492973413));
#32129=CARTESIAN_POINT('Ctrl Pts',(11.5625067173604,-4.00995996944461,4.38146728159866));
#32130=CARTESIAN_POINT('Ctrl Pts',(11.5587504889214,-3.99420842564088,4.37861204937474));
#32131=CARTESIAN_POINT('Origin',(14.8870768733179,-10.,0.));
#32132=CARTESIAN_POINT('',(11.5587511938191,-3.99420842554644,-4.37861112231563));
#32133=CARTESIAN_POINT('',(18.3575990203927,-3.99420842564088,-4.26678755349543));
#32134=CARTESIAN_POINT('Origin',(14.8870768733179,-3.99420842564088,0.));
#32135=CARTESIAN_POINT('',(18.3575990203927,0.,-4.26678755349543));
#32136=CARTESIAN_POINT('',(18.3575990203927,-10.,-4.26678755349543));
#32137=CARTESIAN_POINT('',(11.1121596556826,0.,-4.));
#32138=CARTESIAN_POINT('Origin',(14.8870768733179,0.,0.));
#32139=CARTESIAN_POINT('',(11.1121596556826,0.,4.));
#32140=CARTESIAN_POINT('Ctrl Pts',(11.1121596556826,-1.38777878078145E-16,
4.));
#32141=CARTESIAN_POINT('Ctrl Pts',(11.1121596556826,-0.533653252111662,
4.));
#32142=CARTESIAN_POINT('Ctrl Pts',(10.9882952072323,-1.0734712657027,3.88925687843601));
#32143=CARTESIAN_POINT('Ctrl Pts',(10.6170666685974,-2.04568897841338,3.47761758578428));
#32144=CARTESIAN_POINT('Ctrl Pts',(10.3784032063556,-2.48101536396881,3.17583888552357));
#32145=CARTESIAN_POINT('Ctrl Pts',(9.96544313722852,-3.16971217824285,2.48714207124953));
#32146=CARTESIAN_POINT('Ctrl Pts',(9.75819541135692,-3.47527655703118,2.0509015186475));
#32147=CARTESIAN_POINT('Ctrl Pts',(9.46796099283537,-3.89087901668554,1.06995606602431));
#32148=CARTESIAN_POINT('Ctrl Pts',(9.38707687331794,-4.,0.524242122051539));
#32149=CARTESIAN_POINT('Ctrl Pts',(9.38707687331794,-4.,-0.524242122051539));
#32150=CARTESIAN_POINT('Ctrl Pts',(9.46796099283537,-3.89087901668554,-1.06995606602431));
#32151=CARTESIAN_POINT('Ctrl Pts',(9.75819541135692,-3.47527655703118,-2.0509015186475));
#32152=CARTESIAN_POINT('Ctrl Pts',(9.96544313722852,-3.16971217824285,-2.48714207124953));
#32153=CARTESIAN_POINT('Ctrl Pts',(10.3784032063556,-2.48101536396881,-3.17583888552357));
#32154=CARTESIAN_POINT('Ctrl Pts',(10.6170666685974,-2.04568897841338,-3.47761758578428));
#32155=CARTESIAN_POINT('Ctrl Pts',(10.9882952072323,-1.0734712657027,-3.88925687843601));
#32156=CARTESIAN_POINT('Ctrl Pts',(11.1121596556826,-0.533653252111662,
-4.));
#32157=CARTESIAN_POINT('Ctrl Pts',(11.1121596556826,3.46944695195361E-17,
-4.));
#32158=CARTESIAN_POINT('',(18.3575990203927,0.,4.26678755349543));
#32159=CARTESIAN_POINT('Origin',(14.8870768733179,0.,0.));
#32160=CARTESIAN_POINT('',(18.3575990203927,-10.,4.26678755349543));
#32161=CARTESIAN_POINT('Ctrl Pts',(11.5587480564523,-3.99420842537537,4.37861525003541));
#32162=CARTESIAN_POINT('Ctrl Pts',(11.3626888290799,-4.17260831802453,4.2296270579284));
#32163=CARTESIAN_POINT('Ctrl Pts',(11.1762509051612,-4.34724444370875,4.06742136026345));
#32164=CARTESIAN_POINT('Ctrl Pts',(10.9996449425516,-4.51555528763266,3.89087737077926));
#32165=CARTESIAN_POINT('Ctrl Pts',(10.9109832717729,-4.60005255155271,3.80224681243159));
#32166=CARTESIAN_POINT('Ctrl Pts',(10.8247992487372,-4.68295483008131,3.71000257036262));
#32167=CARTESIAN_POINT('Ctrl Pts',(10.7411172332764,-4.76393373085428,3.61400313546724));
#32168=CARTESIAN_POINT('Ctrl Pts',(10.7349938888345,-4.76985927769047,3.60697847666982));
#32169=CARTESIAN_POINT('Ctrl Pts',(10.7288840068187,-4.77577479692699,3.5999334249579));
#32170=CARTESIAN_POINT('Ctrl Pts',(10.7227876488657,-4.7816801689495,3.5928678430334));
#32171=CARTESIAN_POINT('Ctrl Pts',(10.5986546413389,-4.90192435332469,3.44899966124763));
#32172=CARTESIAN_POINT('Ctrl Pts',(10.4800584128371,-5.01802447019821,3.29654164157823));
#32173=CARTESIAN_POINT('Ctrl Pts',(10.3675209931788,-5.12895882939301,3.13426461014042));
#32174=CARTESIAN_POINT('Ctrl Pts',(10.3643044716539,-5.13212953257135,3.12962644119902));
#32175=CARTESIAN_POINT('Ctrl Pts',(10.3610927721511,-5.13529615364872,3.12497977289136));
#32176=CARTESIAN_POINT('Ctrl Pts',(10.357885971712,-5.13845860697225,3.12032468109803));
#32177=CARTESIAN_POINT('Ctrl Pts',(10.2726922148679,-5.222474212119,2.99665475967357));
#32178=CARTESIAN_POINT('Ctrl Pts',(10.1909180066101,-5.30357974676513,2.86698461435898));
#32179=CARTESIAN_POINT('Ctrl Pts',(10.1140426590526,-5.38013901643824,2.73275773423716));
#32180=CARTESIAN_POINT('Ctrl Pts',(10.0880525528047,-5.40602226271004,2.68737815565284));
#32181=CARTESIAN_POINT('Ctrl Pts',(10.0626225986978,-5.4313856157096,2.64147803497406));
#32182=CARTESIAN_POINT('Ctrl Pts',(10.0378106134104,-5.45616506946334,2.59511401301077));
#32183=CARTESIAN_POINT('Ctrl Pts',(10.0365977316305,-5.45737636100752,2.59284760519095));
#32184=CARTESIAN_POINT('Ctrl Pts',(10.0353862170746,-5.45858636532748,2.59057995299073));
#32185=CARTESIAN_POINT('Ctrl Pts',(10.0341760716815,-5.45979507992655,2.58831105458924));
#32186=CARTESIAN_POINT('Ctrl Pts',(9.95003053478619,-5.5438411288367,2.43054680968724));
#32187=CARTESIAN_POINT('Ctrl Pts',(9.8724914512197,-5.62166228484852,2.26673902468443));
#32188=CARTESIAN_POINT('Ctrl Pts',(9.80219890345532,-5.69242165537877,2.09619946068861));
#32189=CARTESIAN_POINT('Ctrl Pts',(9.78976068958939,-5.70494247318471,2.06602261211724));
#32190=CARTESIAN_POINT('Ctrl Pts',(9.77754944575023,-5.71724209384684,2.03563491622785));
#32191=CARTESIAN_POINT('Ctrl Pts',(9.76556881474159,-5.72931576830717,2.00503247004604));
#32192=CARTESIAN_POINT('Ctrl Pts',(9.76544315633477,-5.72944240259681,2.00471149741701));
#32193=CARTESIAN_POINT('Ctrl Pts',(9.76531752303618,-5.72956901230779,2.00439049834638));
#32194=CARTESIAN_POINT('Ctrl Pts',(9.76519191485892,-5.72969559742598,2.00406947285931));
#32195=CARTESIAN_POINT('Ctrl Pts',(9.71400487072874,-5.78128075829942,1.87324721166454));
#32196=CARTESIAN_POINT('Ctrl Pts',(9.66697657534716,-5.82879541599935,1.73799752918786));
#32197=CARTESIAN_POINT('Ctrl Pts',(9.6250405522746,-5.87123312917844,1.60016514616698));
#32198=CARTESIAN_POINT('Ctrl Pts',(9.60161439240009,-5.89493954148945,1.52316968489148));
#32199=CARTESIAN_POINT('Ctrl Pts',(9.57977711929352,-5.91706181821158,1.44536936046407));
#32200=CARTESIAN_POINT('Ctrl Pts',(9.55968917829128,-5.93742663805485,1.36709188665601));
#32201=CARTESIAN_POINT('Ctrl Pts',(9.55947516461635,-5.93764360155217,1.36625793110865));
#32202=CARTESIAN_POINT('Ctrl Pts',(9.55926134903044,-5.93786036608929,1.36542391969325));
#32203=CARTESIAN_POINT('Ctrl Pts',(9.55904773172286,-5.93807693146144,1.36458985278468));
#32204=CARTESIAN_POINT('Ctrl Pts',(9.50331705704126,-5.99457672747216,1.1469899210633));
#32205=CARTESIAN_POINT('Ctrl Pts',(9.46041989832733,-6.0381883908994,0.924289620191035));
#32206=CARTESIAN_POINT('Ctrl Pts',(9.43130753977526,-6.06780345239864,0.696118554534736));
#32207=CARTESIAN_POINT('Ctrl Pts',(9.43114806151225,-6.06796568448157,0.694868627458047));
#32208=CARTESIAN_POINT('Ctrl Pts',(9.43098899634983,-6.06812749717018,0.693618531424424));
#32209=CARTESIAN_POINT('Ctrl Pts',(9.43083034447406,-6.06828889025085,0.69236826651728));
#32210=CARTESIAN_POINT('Ctrl Pts',(9.41547288739991,-6.08391169519064,0.571342974191852));
#32211=CARTESIAN_POINT('Ctrl Pts',(9.40406058123609,-6.09552882987824,0.448312367480381));
#32212=CARTESIAN_POINT('Ctrl Pts',(9.39675231043817,-6.10297030911209,0.324915545562507));
#32213=CARTESIAN_POINT('Ctrl Pts',(9.39030112011018,-6.10953908580177,0.215990136793151));
#32214=CARTESIAN_POINT('Ctrl Pts',(9.38704741662975,-6.11285457215368,0.106780944007842));
#32215=CARTESIAN_POINT('Ctrl Pts',(9.38707711882443,-6.11282361448583,-0.00157937270664588));
#32216=CARTESIAN_POINT('Ctrl Pts',(9.38707738015422,-6.11282334210997,-0.00253276283819925));
#32217=CARTESIAN_POINT('Ctrl Pts',(9.38707789550786,-6.1128228109299,-0.00348609118645972));
#32218=CARTESIAN_POINT('Ctrl Pts',(9.38707866494222,-6.11282202088418,-0.00443935704251815));
#32219=CARTESIAN_POINT('Ctrl Pts',(9.3872654421285,-6.11263024037226,-0.235840921054131));
#32220=CARTESIAN_POINT('Ctrl Pts',(9.40199748120688,-6.09761913563677,-0.465515426606816));
#32221=CARTESIAN_POINT('Ctrl Pts',(9.4309684633591,-6.06814824803631,-0.693455868487982));
#32222=CARTESIAN_POINT('Ctrl Pts',(9.43106885022933,-6.06804612895199,-0.694245701136398));
#32223=CARTESIAN_POINT('Ctrl Pts',(9.43116940824751,-6.06794383609246,-0.695035514567625));
#32224=CARTESIAN_POINT('Ctrl Pts',(9.43127013739879,-6.06784136947459,-0.695825308751845));
#32225=CARTESIAN_POINT('Ctrl Pts',(9.44755402646091,-6.05127660131423,-0.823503549992644));
#32226=CARTESIAN_POINT('Ctrl Pts',(9.46849384706743,-6.02998478850161,-0.951092004927493));
#32227=CARTESIAN_POINT('Ctrl Pts',(9.49358748617142,-6.00450023692484,-1.07683420677694));
#32228=CARTESIAN_POINT('Ctrl Pts',(9.51331996418398,-5.98446036341089,-1.17571206275323));
#32229=CARTESIAN_POINT('Ctrl Pts',(9.53562010983275,-5.96182877448762,-1.27344794850474));
#32230=CARTESIAN_POINT('Ctrl Pts',(9.56023113615348,-5.93687782718841,-1.36920204958066));
#32231=CARTESIAN_POINT('Ctrl Pts',(9.56048990352749,-5.93661548578795,-1.37020883560263));
#32232=CARTESIAN_POINT('Ctrl Pts',(9.56074892743608,-5.93635288702437,-1.37121540719265));
#32233=CARTESIAN_POINT('Ctrl Pts',(9.56100820760137,-5.93609003119388,-1.37222176345421));
#32234=CARTESIAN_POINT('Ctrl Pts',(9.61696238254866,-5.87936420680227,-1.58939932601352));
#32235=CARTESIAN_POINT('Ctrl Pts',(9.68492647384057,-5.81058800718736,-1.7984972507641));
#32236=CARTESIAN_POINT('Ctrl Pts',(9.76373024102914,-5.73116881967472,-2.00032985222453));
#32237=CARTESIAN_POINT('Ctrl Pts',(9.76456463201257,-5.7303279124905,-2.00246689857179));
#32238=CARTESIAN_POINT('Ctrl Pts',(9.76540023933697,-5.72948581132656,-2.00460313210208));
#32239=CARTESIAN_POINT('Ctrl Pts',(9.76623706163906,-5.72864251781373,-2.0067385537552));
#32240=CARTESIAN_POINT('Ctrl Pts',(9.82523364578579,-5.66918970857808,-2.15728734163231));
#32241=CARTESIAN_POINT('Ctrl Pts',(9.89067957083013,-5.60339936653193,-2.30450833756059));
#32242=CARTESIAN_POINT('Ctrl Pts',(9.96126858557544,-5.53271401884161,-2.4466727459975));
#32243=CARTESIAN_POINT('Ctrl Pts',(9.98467942415214,-5.50927123145484,-2.49382155561435));
#32244=CARTESIAN_POINT('Ctrl Pts',(10.0086561730407,-5.48528979005206,-2.54041446084365));
#32245=CARTESIAN_POINT('Ctrl Pts',(10.0331518093073,-5.46082159602852,-2.58638921905928));
#32246=CARTESIAN_POINT('Ctrl Pts',(10.0352622179174,-5.45871355169039,-2.59035015008101));
#32247=CARTESIAN_POINT('Ctrl Pts',(10.0373764572102,-5.45660191865752,-2.59430645369377));
#32248=CARTESIAN_POINT('Ctrl Pts',(10.0394944974403,-5.45448672989252,-2.59825809134046));
#32249=CARTESIAN_POINT('Ctrl Pts',(10.1231772780924,-5.37091660929666,-2.75438544987707));
#32250=CARTESIAN_POINT('Ctrl Pts',(10.2123532673795,-5.28219670560045,-2.90302025346162));
#32251=CARTESIAN_POINT('Ctrl Pts',(10.3066428918801,-5.18899936326121,-3.04491648351723));
#32252=CARTESIAN_POINT('Ctrl Pts',(10.4047692317532,-5.09200975132797,-3.19258657734662));
#32253=CARTESIAN_POINT('Ctrl Pts',(10.5084338580352,-4.99017075072625,-3.33295843771009));
#32254=CARTESIAN_POINT('Ctrl Pts',(10.6172356637028,-4.88420776535908,-3.46684409098579));
#32255=CARTESIAN_POINT('Ctrl Pts',(10.6505136862934,-4.85179802179666,-3.50779423668353));
#32256=CARTESIAN_POINT('Ctrl Pts',(10.6842724713102,-4.81900226877546,-3.54813734782343));
#32257=CARTESIAN_POINT('Ctrl Pts',(10.718501004134,-4.78584072941129,-3.58789601986351));
#32258=CARTESIAN_POINT('Ctrl Pts',(10.7258311426537,-4.77873909060255,-3.59641045356464));
#32259=CARTESIAN_POINT('Ctrl Pts',(10.7331821298285,-4.77162136370932,-3.60489727595804));
#32260=CARTESIAN_POINT('Ctrl Pts',(10.7405539922153,-4.76448761189709,-3.6133568876269));
#32261=CARTESIAN_POINT('Ctrl Pts',(10.8109577635415,-4.69635787684114,-3.69414903134668));
#32262=CARTESIAN_POINT('Ctrl Pts',(10.8832920761415,-4.62673602708103,-3.77233650058384));
#32263=CARTESIAN_POINT('Ctrl Pts',(10.9573999400201,-4.55592983802426,-3.84797903420149));
#32264=CARTESIAN_POINT('Ctrl Pts',(11.0332070572439,-4.48350010124507,-3.92535601031363));
#32265=CARTESIAN_POINT('Ctrl Pts',(11.1108707017101,-4.40982991477362,-4.00007045807862));
#32266=CARTESIAN_POINT('Ctrl Pts',(11.1902510794477,-4.33523070780175,-4.07214227964421));
#32267=CARTESIAN_POINT('Ctrl Pts',(11.2682864139836,-4.26189553054412,-4.14299289621692));
#32268=CARTESIAN_POINT('Ctrl Pts',(11.3479816279103,-4.18766133326008,-4.21128986378364));
#32269=CARTESIAN_POINT('Ctrl Pts',(11.4292191118081,-4.11282480171223,-4.27700572216152));
#32270=CARTESIAN_POINT('Ctrl Pts',(11.4719750782119,-4.07343771000138,-4.31159252739222));
#32271=CARTESIAN_POINT('Ctrl Pts',(11.515158434596,-4.03388389452131,-4.34546356908915));
#32272=CARTESIAN_POINT('Ctrl Pts',(11.5587526034551,-3.99420842547088,-4.37860926807613));
#32273=CARTESIAN_POINT('Origin',(-3.88784034431744,0.,0.));
#32274=CARTESIAN_POINT('',(-2.88899111509131,-7.40661556618246E-16,6.04796058042142));
#32275=CARTESIAN_POINT('Origin',(-2.88899111509131,0.,0.));
#32276=CARTESIAN_POINT('',(-3.88784034431744,-6.0599836255502E-16,4.94835215326525));
#32277=CARTESIAN_POINT('',(-3.88784034431744,-6.0599836255502E-16,4.94835215326525));
#32278=CARTESIAN_POINT('Origin',(-3.88784034431744,0.,0.));
#32279=CARTESIAN_POINT('Origin',(18.3245838861624,0.,0.));
#32280=CARTESIAN_POINT('',(18.3706375907924,0.,-4.25614904904291));
#32281=CARTESIAN_POINT('',(18.5421134565937,0.,-4.27463759471298));
#32282=CARTESIAN_POINT('Origin',(18.3245838861624,0.,-5.48772230081581));
#32283=CARTESIAN_POINT('',(18.9788234605247,-4.08475030728679,-5.09745204146194));
#32284=CARTESIAN_POINT('Ctrl Pts',(18.5421134565937,-4.25668091127711E-16,
-4.27463759471298));
#32285=CARTESIAN_POINT('Ctrl Pts',(18.5421134565937,-0.0254801014594758,
-4.27463759471298));
#32286=CARTESIAN_POINT('Ctrl Pts',(18.5445357600052,-0.0504618671715304,
-4.27483896810787));
#32287=CARTESIAN_POINT('Ctrl Pts',(18.5488507525854,-0.0749847941031531,
-4.27520750677706));
#32288=CARTESIAN_POINT('Ctrl Pts',(18.5549572286634,-0.109689063899206,
-4.27572905403939));
#32289=CARTESIAN_POINT('Ctrl Pts',(18.5648536938036,-0.143474544424252,
-4.27659263523378));
#32290=CARTESIAN_POINT('Ctrl Pts',(18.577017371859,-0.176443360724415,-4.27778034521236));
#32291=CARTESIAN_POINT('Ctrl Pts',(18.5859098337359,-0.200545769612747,
-4.27864864061259));
#32292=CARTESIAN_POINT('Ctrl Pts',(18.5960132886523,-0.224211738802833,
-4.2796923434056));
#32293=CARTESIAN_POINT('Ctrl Pts',(18.6067345431864,-0.247476011988283,
-4.28087311968421));
#32294=CARTESIAN_POINT('Ctrl Pts',(18.6106785062611,-0.256034099487255,
-4.28130748471373));
#32295=CARTESIAN_POINT('Ctrl Pts',(18.6147061344625,-0.264537763086523,
-4.2817599332196));
#32296=CARTESIAN_POINT('Ctrl Pts',(18.6187881934998,-0.272988456681822,
-4.28222671824238));
#32297=CARTESIAN_POINT('Ctrl Pts',(18.6338157474098,-0.304098553920046,
-4.28394512481861));
#32298=CARTESIAN_POINT('Ctrl Pts',(18.6497999181611,-0.334819746905005,
-4.28589352869452));
#32299=CARTESIAN_POINT('Ctrl Pts',(18.6663913361296,-0.365265144948759,
-4.28810690858487));
#32300=CARTESIAN_POINT('Ctrl Pts',(18.6822196269575,-0.394310197971121,
-4.29021848341734));
#32301=CARTESIAN_POINT('Ctrl Pts',(18.6986002223778,-0.423104522276839,
-4.29257138621942));
#32302=CARTESIAN_POINT('Ctrl Pts',(18.7152343269478,-0.451742333789593,
-4.29514932713806));
#32303=CARTESIAN_POINT('Ctrl Pts',(18.7288317921048,-0.475152168841498,
-4.29725665198207));
#32304=CARTESIAN_POINT('Ctrl Pts',(18.742598638901,-0.498457416161126,-4.29951352128347));
#32305=CARTESIAN_POINT('Ctrl Pts',(18.7563766796154,-0.521705510096399,
-4.30188582063063));
#32306=CARTESIAN_POINT('Ctrl Pts',(18.783169802229,-0.566914335084774,-4.30649905328121));
#32307=CARTESIAN_POINT('Ctrl Pts',(18.8101446723159,-0.611979171936971,
-4.31158867889594));
#32308=CARTESIAN_POINT('Ctrl Pts',(18.8370689932334,-0.657009298536488,
-4.31718836948623));
#32309=CARTESIAN_POINT('Ctrl Pts',(18.8638321278848,-0.701769845896118,
-4.32275453673455));
#32310=CARTESIAN_POINT('Ctrl Pts',(18.890544823512,-0.746496520158024,-4.3288246153777));
#32311=CARTESIAN_POINT('Ctrl Pts',(18.9169838610535,-0.791287166948651,
-4.33538155269578));
#32312=CARTESIAN_POINT('Ctrl Pts',(18.943298883484,-0.835867718457729,-4.34190773400361));
#32313=CARTESIAN_POINT('Ctrl Pts',(18.9693423170444,-0.880512000020209,
-4.34891600802757));
#32314=CARTESIAN_POINT('Ctrl Pts',(18.9949063476124,-0.925301239209109,
-4.35634180429196));
#32315=CARTESIAN_POINT('Ctrl Pts',(19.0109806429501,-0.953464069665662,
-4.36101103835323));
#32316=CARTESIAN_POINT('Ctrl Pts',(19.0268656680106,-0.981683884269773,
-4.36584439788146));
#32317=CARTESIAN_POINT('Ctrl Pts',(19.042513570575,-1.00997688847436,-4.37081681177666));
#32318=CARTESIAN_POINT('Ctrl Pts',(19.0798137917417,-1.07741949363883,-4.38266965513763));
#32319=CARTESIAN_POINT('Ctrl Pts',(19.1158787124396,-1.14523365849758,-4.39540379894711));
#32320=CARTESIAN_POINT('Ctrl Pts',(19.1504383167282,-1.21359345665619,-4.4089470513481));
#32321=CARTESIAN_POINT('Ctrl Pts',(19.1844668878412,-1.28090285735068,-4.42228220193544));
#32322=CARTESIAN_POINT('Ctrl Pts',(19.2170359214768,-1.34874153614133,-4.43640163180863));
#32323=CARTESIAN_POINT('Ctrl Pts',(19.2478784152531,-1.41724208592662,-4.45119997195958));
#32324=CARTESIAN_POINT('Ctrl Pts',(19.2618719954876,-1.44832154229253,-4.45791414240713));
#32325=CARTESIAN_POINT('Ctrl Pts',(19.2755100453659,-1.47953675967748,-4.46476758171775));
#32326=CARTESIAN_POINT('Ctrl Pts',(19.2887671097419,-1.51089754629334,-4.47174804387616));
#32327=CARTESIAN_POINT('Ctrl Pts',(19.3157307639414,-1.57468251268946,-4.48594566428848));
#32328=CARTESIAN_POINT('Ctrl Pts',(19.3411921421037,-1.63922105464934,-4.50071861138956));
#32329=CARTESIAN_POINT('Ctrl Pts',(19.3648781089758,-1.70442847903499,-4.51596285581109));
#32330=CARTESIAN_POINT('Ctrl Pts',(19.3879193855577,-1.76786107220608,-4.53079217875556));
#32331=CARTESIAN_POINT('Ctrl Pts',(19.4092802005646,-1.83192674775908,-4.54606702186589));
#32332=CARTESIAN_POINT('Ctrl Pts',(19.4287217645248,-1.89650177828534,-4.5616800383172));
#32333=CARTESIAN_POINT('Ctrl Pts',(19.4427734845,-1.94317447643887,-4.57296461066907));
#32334=CARTESIAN_POINT('Ctrl Pts',(19.4558228421615,-1.9901123111244,-4.58442557886488));
#32335=CARTESIAN_POINT('Ctrl Pts',(19.4677856588679,-2.03725270625742,-4.59602059784627));
#32336=CARTESIAN_POINT('Ctrl Pts',(19.4836157479168,-2.09963238414392,-4.61136398958295));
#32337=CARTESIAN_POINT('Ctrl Pts',(19.4975218504262,-2.16228822832006,-4.62690576465906));
#32338=CARTESIAN_POINT('Ctrl Pts',(19.5093789068896,-2.22527395400374,-4.64262367122429));
#32339=CARTESIAN_POINT('Ctrl Pts',(19.5206604386916,-2.28520244212082,-4.65757865295381));
#32340=CARTESIAN_POINT('Ctrl Pts',(19.5300868182461,-2.34542993100449,-4.67269369206331));
#32341=CARTESIAN_POINT('Ctrl Pts',(19.5375083329815,-2.40599268770172,-4.68793464693561));
#32342=CARTESIAN_POINT('Ctrl Pts',(19.5447205451536,-2.46484744533578,-4.70274577433533));
#32343=CARTESIAN_POINT('Ctrl Pts',(19.5500392215662,-2.52401927226447,-4.71767635525021));
#32344=CARTESIAN_POINT('Ctrl Pts',(19.5532886451223,-2.58352585445992,-4.73267227407408));
#32345=CARTESIAN_POINT('Ctrl Pts',(19.5568715014676,-2.64913857989318,-4.74920696768458));
#32346=CARTESIAN_POINT('Ctrl Pts',(19.5579208431573,-2.71488993281246,-4.76576752417364));
#32347=CARTESIAN_POINT('Ctrl Pts',(19.5562274234509,-2.78054074813488,-4.78226180213361));
#32348=CARTESIAN_POINT('Ctrl Pts',(19.5545894883089,-2.84404052737642,-4.79821564831301));
#32349=CARTESIAN_POINT('Ctrl Pts',(19.5503851390046,-2.90744624410649,-4.81410756418141));
#32350=CARTESIAN_POINT('Ctrl Pts',(19.543432946332,-2.97049514836484,-4.82984508554704));
#32351=CARTESIAN_POINT('Ctrl Pts',(19.537295918086,-3.0261513887096,-4.84373733763073));
#32352=CARTESIAN_POINT('Ctrl Pts',(19.5290174995114,-3.08152901217754,-4.85750921071767));
#32353=CARTESIAN_POINT('Ctrl Pts',(19.5184828236628,-3.13641568626229,-4.87109011242972));
#32354=CARTESIAN_POINT('Ctrl Pts',(19.5095221706226,-3.18310155017265,-4.88264184406006));
#32355=CARTESIAN_POINT('Ctrl Pts',(19.4989688849651,-3.22928780844808,-4.89398417428052));
#32356=CARTESIAN_POINT('Ctrl Pts',(19.4867363354049,-3.27496260554755,-4.90515615271697));
#32357=CARTESIAN_POINT('Ctrl Pts',(19.4747569202957,-3.31969223053607,-4.91609694364712));
#32358=CARTESIAN_POINT('Ctrl Pts',(19.461166645143,-3.36393186154866,-4.92687481197273));
#32359=CARTESIAN_POINT('Ctrl Pts',(19.4458481150729,-3.40765453681482,-4.93749794545092));
#32360=CARTESIAN_POINT('Ctrl Pts',(19.4309480706269,-3.45018275602269,-4.94783086644636));
#32361=CARTESIAN_POINT('Ctrl Pts',(19.4144124535007,-3.49222233510551,-4.958017738087));
#32362=CARTESIAN_POINT('Ctrl Pts',(19.3961048908036,-3.53372627849561,-4.96803313457627));
#32363=CARTESIAN_POINT('Ctrl Pts',(19.3777973281065,-3.57523022188571,-4.97804853106554));
#32364=CARTESIAN_POINT('Ctrl Pts',(19.3577173695828,-3.61619911705965,-4.98789295307204));
#32365=CARTESIAN_POINT('Ctrl Pts',(19.3357063971287,-3.65655558431263,-4.99750105264302));
#32366=CARTESIAN_POINT('Ctrl Pts',(19.313266779319,-3.69769796015238,-5.00729626195055));
#32367=CARTESIAN_POINT('Ctrl Pts',(19.289134021862,-3.73764489679991,-5.01669780151543));
#32368=CARTESIAN_POINT('Ctrl Pts',(19.2632223927464,-3.7762889522877,-5.02575304016386));
#32369=CARTESIAN_POINT('Ctrl Pts',(19.2390742535079,-3.8123029762803,-5.03419199870034));
#32370=CARTESIAN_POINT('Ctrl Pts',(19.2133802940762,-3.84718564933888,-5.04233026248691));
#32371=CARTESIAN_POINT('Ctrl Pts',(19.1860503642663,-3.8808244610573,-5.05017035603905));
#32372=CARTESIAN_POINT('Ctrl Pts',(19.1594485534184,-3.91356707374257,-5.05780157526114));
#32373=CARTESIAN_POINT('Ctrl Pts',(19.1312961252711,-3.94513151564625,-5.06515054788063));
#32374=CARTESIAN_POINT('Ctrl Pts',(19.1014999739291,-3.9753850188093,-5.0721818065022));
#32375=CARTESIAN_POINT('Ctrl Pts',(19.0728862687923,-4.00443792597597,-5.07893403294343));
#32376=CARTESIAN_POINT('Ctrl Pts',(19.0427560661447,-4.03228200530944,-5.08539335384616));
#32377=CARTESIAN_POINT('Ctrl Pts',(19.0110269646178,-4.05876964694868,-5.09149074847995));
#32378=CARTESIAN_POINT('Ctrl Pts',(19.0004703578505,-4.0675823647227,-5.09351941599201));
#32379=CARTESIAN_POINT('Ctrl Pts',(18.9897368016208,-4.07624466766795,-5.095507695138));
#32380=CARTESIAN_POINT('Ctrl Pts',(18.9788234605247,-4.08475030728679,-5.09745204146194));
#32381=CARTESIAN_POINT('',(18.9788234605247,-4.08475030728679,5.09745204146194));
#32382=CARTESIAN_POINT('Origin',(18.9788234605247,0.,0.));
#32383=CARTESIAN_POINT('',(18.5421134565937,0.,4.27463759471298));
#32384=CARTESIAN_POINT('Ctrl Pts',(18.9788234605247,-4.08475030728679,5.09745204146194));
#32385=CARTESIAN_POINT('Ctrl Pts',(19.0092155017241,-4.06106335867525,5.09203732445985));
#32386=CARTESIAN_POINT('Ctrl Pts',(19.038201878942,-4.03614678048446,5.08630814962051));
#32387=CARTESIAN_POINT('Ctrl Pts',(19.0658854085647,-4.01010768196352,5.08030731363521));
#32388=CARTESIAN_POINT('Ctrl Pts',(19.0945031333629,-3.98318988045413,5.07410397630336));
#32389=CARTESIAN_POINT('Ctrl Pts',(19.1217292974,-3.95507228369758,5.06761017514692));
#32390=CARTESIAN_POINT('Ctrl Pts',(19.1476684840898,-3.92584011263657,5.0608292638313));
#32391=CARTESIAN_POINT('Ctrl Pts',(19.1587650009721,-3.91333489095928,5.05792845981647));
#32392=CARTESIAN_POINT('Ctrl Pts',(19.1696258235112,-3.90062531636491,5.05497459316725));
#32393=CARTESIAN_POINT('Ctrl Pts',(19.180258194112,-3.88771648264067,5.05196571294776));
#32394=CARTESIAN_POINT('Ctrl Pts',(19.2038753205281,-3.85904276824554,5.045282245339));
#32395=CARTESIAN_POINT('Ctrl Pts',(19.2264219802684,-3.82928334263606,5.03832874515852));
#32396=CARTESIAN_POINT('Ctrl Pts',(19.2477875023842,-3.79870511095283,5.03114432286621));
#32397=CARTESIAN_POINT('Ctrl Pts',(19.2693156963375,-3.76789406412439,5.02390520014726));
#32398=CARTESIAN_POINT('Ctrl Pts',(19.2896444858868,-3.73625219157716,5.01643186588051));
#32399=CARTESIAN_POINT('Ctrl Pts',(19.3087047767471,-3.70405870503921,5.0087932128783));
#32400=CARTESIAN_POINT('Ctrl Pts',(19.3184086433773,-3.68766854069105,5.00490426540574));
#32401=CARTESIAN_POINT('Ctrl Pts',(19.3277844439617,-3.67113545045191,5.00097290629788));
#32402=CARTESIAN_POINT('Ctrl Pts',(19.3368275939036,-3.65449625972552,4.99701072297555));
#32403=CARTESIAN_POINT('Ctrl Pts',(19.363374077786,-3.60565133165635,4.98537959484204));
#32404=CARTESIAN_POINT('Ctrl Pts',(19.3873130954724,-3.55545669304448,4.97334289549462));
#32405=CARTESIAN_POINT('Ctrl Pts',(19.4087322482119,-3.50426728284812,4.96099350117674));
#32406=CARTESIAN_POINT('Ctrl Pts',(19.4306743089924,-3.45182818016717,4.94834261978939));
#32407=CARTESIAN_POINT('Ctrl Pts',(19.4499725786457,-3.39834527030435,4.93536346761216));
#32408=CARTESIAN_POINT('Ctrl Pts',(19.4667506470085,-3.34415611304767,4.92213926982721));
#32409=CARTESIAN_POINT('Ctrl Pts',(19.4841244237279,-3.28804295994605,4.9084455445043));
#32410=CARTESIAN_POINT('Ctrl Pts',(19.4987964466969,-3.23117263090285,4.89448894356967));
#32411=CARTESIAN_POINT('Ctrl Pts',(19.5109258361256,-3.17387129428592,4.88034611034631));
#32412=CARTESIAN_POINT('Ctrl Pts',(19.5139266235123,-3.15969505489859,4.87684720087532));
#32413=CARTESIAN_POINT('Ctrl Pts',(19.5167718648232,-3.14549220605671,4.87333682487201));
#32414=CARTESIAN_POINT('Ctrl Pts',(19.5194641043032,-3.13126724135225,4.86981601487401));
#32415=CARTESIAN_POINT('Ctrl Pts',(19.5310219267275,-3.07019926531775,4.85470112741758));
#32416=CARTESIAN_POINT('Ctrl Pts',(19.5397754782162,-3.00866440890858,4.83935864683886));
#32417=CARTESIAN_POINT('Ctrl Pts',(19.5459099142417,-2.94691930253355,4.82389985356588));
#32418=CARTESIAN_POINT('Ctrl Pts',(19.5522227928369,-2.88337811329133,4.80799138459591));
#32419=CARTESIAN_POINT('Ctrl Pts',(19.5557625400972,-2.81961415152491,4.7919596033858));
#32420=CARTESIAN_POINT('Ctrl Pts',(19.5567380782345,-2.75585562629362,4.77590586845312));
#32421=CARTESIAN_POINT('Ctrl Pts',(19.5577584028666,-2.68916997730747,4.75911511413825));
#32422=CARTESIAN_POINT('Ctrl Pts',(19.5559742312122,-2.62249021315083,4.74230020891914));
#32423=CARTESIAN_POINT('Ctrl Pts',(19.5516233603138,-2.55602310574085,4.72555767462613));
#32424=CARTESIAN_POINT('Ctrl Pts',(19.5471598377419,-2.48783504842201,4.70838164677534));
#32425=CARTESIAN_POINT('Ctrl Pts',(19.5399954701845,-2.41987049650095,4.69128154228306));
#32426=CARTESIAN_POINT('Ctrl Pts',(19.5303775138833,-2.35229992639511,4.6743446041456));
#32427=CARTESIAN_POINT('Ctrl Pts',(19.520376925709,-2.28204119125675,4.6567338625344));
#32428=CARTESIAN_POINT('Ctrl Pts',(19.507724084395,-2.21220816070646,4.63929926101361));
#32429=CARTESIAN_POINT('Ctrl Pts',(19.492679467708,-2.14294033361043,4.62212469053316));
#32430=CARTESIAN_POINT('Ctrl Pts',(19.4850149126374,-2.10765149332649,4.61337501987018));
#32431=CARTESIAN_POINT('Ctrl Pts',(19.4767292665588,-2.0725085539897,4.60469264187981));
#32432=CARTESIAN_POINT('Ctrl Pts',(19.4678548462165,-2.03752539429306,4.5960876712563));
#32433=CARTESIAN_POINT('Ctrl Pts',(19.4506703711719,-1.96978381663498,4.5794249600892));
#32434=CARTESIAN_POINT('Ctrl Pts',(19.4312143025218,-1.90239275960969,4.56299625837018));
#32435=CARTESIAN_POINT('Ctrl Pts',(19.4097043313689,-1.83546262513185,4.54693533472414));
#32436=CARTESIAN_POINT('Ctrl Pts',(19.3868675723589,-1.76440407555393,4.52988373385595));
#32437=CARTESIAN_POINT('Ctrl Pts',(19.3617159606843,-1.69386543536571,4.5132472326653));
#32438=CARTESIAN_POINT('Ctrl Pts',(19.334527787239,-1.62391968717625,4.49717291690614));
#32439=CARTESIAN_POINT('Ctrl Pts',(19.3080958649913,-1.55591951123851,4.48154571542506));
#32440=CARTESIAN_POINT('Ctrl Pts',(19.2797395402235,-1.48847914543718,4.46645016856151));
#32441=CARTESIAN_POINT('Ctrl Pts',(19.2497252658693,-1.42161421705033,4.45200331335871));
#32442=CARTESIAN_POINT('Ctrl Pts',(19.2184228711861,-1.35187965161869,4.43693644357022));
#32443=CARTESIAN_POINT('Ctrl Pts',(19.1853175219329,-1.28277087816504,4.42257571144363));
#32444=CARTESIAN_POINT('Ctrl Pts',(19.1507173950585,-1.21425305164681,4.40902684453694));
#32445=CARTESIAN_POINT('Ctrl Pts',(19.1161172681841,-1.14573522512858,4.39547797763025));
#32446=CARTESIAN_POINT('Ctrl Pts',(19.0800227461583,-1.07780776258487,4.38274130761694));
#32447=CARTESIAN_POINT('Ctrl Pts',(19.0427420848227,-1.01039009749801,4.37088944250479));
#32448=CARTESIAN_POINT('Ctrl Pts',(19.0176862009639,-0.965079496078312,
4.36292394658491));
#32449=CARTESIAN_POINT('Ctrl Pts',(18.9920359319277,-0.919985408305112,
4.35532184851541));
#32450=CARTESIAN_POINT('Ctrl Pts',(18.9659876672824,-0.875027301247306,
4.34817500505906));
#32451=CARTESIAN_POINT('Ctrl Pts',(18.9398815492249,-0.829969341860113,
4.34101228840401));
#32452=CARTESIAN_POINT('Ctrl Pts',(18.9133761474955,-0.785047651405376,
4.33430711611102));
#32453=CARTESIAN_POINT('Ctrl Pts',(18.8866851821932,-0.740163271093601,
4.32810525027266));
#32454=CARTESIAN_POINT('Ctrl Pts',(18.8597891825343,-0.694934098454789,
4.32185574301118));
#32455=CARTESIAN_POINT('Ctrl Pts',(18.8327052521153,-0.649742429280504,
4.31611747411665));
#32456=CARTESIAN_POINT('Ctrl Pts',(18.8056609345573,-0.604474127390862,
4.31088651744545));
#32457=CARTESIAN_POINT('Ctrl Pts',(18.789219980108,-0.576954331863708,4.30770648081951));
#32458=CARTESIAN_POINT('Ctrl Pts',(18.7727938031056,-0.54940598728245,4.30471292813371));
#32459=CARTESIAN_POINT('Ctrl Pts',(18.7564339386911,-0.521802123955709,
4.30189568020001));
#32460=CARTESIAN_POINT('Ctrl Pts',(18.7397027696494,-0.49357176141591,4.29901449181013));
#32461=CARTESIAN_POINT('Ctrl Pts',(18.7229895518091,-0.465269352172632,
4.29630414918437));
#32462=CARTESIAN_POINT('Ctrl Pts',(18.7065689069815,-0.436780695224228,
4.29382139179048));
#32463=CARTESIAN_POINT('Ctrl Pts',(18.6895291685526,-0.407217954681067,
4.2912450291069));
#32464=CARTESIAN_POINT('Ctrl Pts',(18.6728048477287,-0.377454401795733,
4.28891382372324));
#32465=CARTESIAN_POINT('Ctrl Pts',(18.6567126558758,-0.34735464947781,4.28683470028683));
#32466=CARTESIAN_POINT('Ctrl Pts',(18.6435340824926,-0.322704695117279,
4.28513201857449));
#32467=CARTESIAN_POINT('Ctrl Pts',(18.6307797349848,-0.297829040646783,
4.28359715999337));
#32468=CARTESIAN_POINT('Ctrl Pts',(18.6186255330937,-0.272651611164468,
4.28220812332119));
#32469=CARTESIAN_POINT('Ctrl Pts',(18.6073623729794,-0.249319974742047,
4.28092091889726));
#32470=CARTESIAN_POINT('Ctrl Pts',(18.5965521051593,-0.225577884414913,
4.27975640143456));
#32471=CARTESIAN_POINT('Ctrl Pts',(18.5867835955735,-0.201439120566317,
4.27876353217638));
#32472=CARTESIAN_POINT('Ctrl Pts',(18.5737591691624,-0.169254727375367,
4.2774397322174));
#32473=CARTESIAN_POINT('Ctrl Pts',(18.5625877203779,-0.13636500536244,4.2764190207263));
#32474=CARTESIAN_POINT('Ctrl Pts',(18.5546757430905,-0.102787459871969,
4.27572220356722));
#32475=CARTESIAN_POINT('Ctrl Pts',(18.5488806896841,-0.0781939022432147,
4.27521182638783));
#32476=CARTESIAN_POINT('Ctrl Pts',(18.5448346783279,-0.0532311433030454,
4.27487102240903));
#32477=CARTESIAN_POINT('Ctrl Pts',(18.5430852251124,-0.0279031173504605,
4.27472118600104));
#32478=CARTESIAN_POINT('Ctrl Pts',(18.5424461526085,-0.0186508293669923,
4.27466645099722));
#32479=CARTESIAN_POINT('Ctrl Pts',(18.5421134565937,-0.00934977220112235,
4.27463759471298));
#32480=CARTESIAN_POINT('Ctrl Pts',(18.5421134565937,0.,4.27463759471298));
#32481=CARTESIAN_POINT('',(18.3706375907924,0.,4.25614904904291));
#32482=CARTESIAN_POINT('Origin',(18.3245838861624,0.,5.48772230081581));
#32483=CARTESIAN_POINT('Origin',(18.3706375907924,0.,0.));
#32484=CARTESIAN_POINT('Origin',(14.8870768733179,0.,0.));
#32485=CARTESIAN_POINT('Origin',(14.8870768733179,0.,0.));
#32486=CARTESIAN_POINT('Origin',(11.1121596556826,0.,0.));
#32487=CARTESIAN_POINT('Origin',(14.8870768733179,0.,0.));
#32488=CARTESIAN_POINT('Origin',(-60.4312629272455,0.,0.));
#32489=CARTESIAN_POINT('',(-3.88784034431744,-4.89858719658941E-16,-4.));
#32490=CARTESIAN_POINT('',(-60.4312629272455,-4.89858719658941E-16,-4.));
#32491=CARTESIAN_POINT('Origin',(-3.88784034431744,0.,0.));
#32492=CARTESIAN_POINT('Origin',(11.1121596556826,0.,0.));
#32493=CARTESIAN_POINT('',(11.1121596556826,-8.22991738629016E-16,6.72023753462643));
#32494=CARTESIAN_POINT('Origin',(11.1121596556826,0.,0.));
#32495=CARTESIAN_POINT('',(11.1121596556826,-8.22991738629016E-16,6.72023753462643));
#32496=CARTESIAN_POINT('',(11.1121596556826,-4.27128032554705,-5.18823254127999));
#32497=CARTESIAN_POINT('Origin',(11.1121596556826,0.,0.));
#32498=CARTESIAN_POINT('',(11.1585526803519,-4.38134327770265,-5.09856534401068));
#32499=CARTESIAN_POINT('Ctrl Pts',(11.1121596556826,-4.27128032554706,-5.18823254127999));
#32500=CARTESIAN_POINT('Ctrl Pts',(11.1121596556826,-4.27665349298167,-5.18380901088371));
#32501=CARTESIAN_POINT('Ctrl Pts',(11.1124205603573,-4.2820265275568,-5.17938779583192));
#32502=CARTESIAN_POINT('Ctrl Pts',(11.1153502651155,-4.31100162102884,-5.15556504699343));
#32503=CARTESIAN_POINT('Ctrl Pts',(11.1231194250036,-4.33370705720515,-5.13696310729952));
#32504=CARTESIAN_POINT('Ctrl Pts',(11.143213732739,-4.36424955048543,-5.11225066055275));
#32505=CARTESIAN_POINT('Ctrl Pts',(11.1504180869028,-4.37306471988177,-5.10516435342262));
#32506=CARTESIAN_POINT('Ctrl Pts',(11.1585526803519,-4.38134327770264,-5.09856534401069));
#32507=CARTESIAN_POINT('Ctrl Pts',(11.1585526803519,-4.38134327770267,-5.09856534401067));
#32508=CARTESIAN_POINT('Ctrl Pts',(10.8280078030872,-4.68201126458796,-4.8192662818435));
#32509=CARTESIAN_POINT('Ctrl Pts',(10.5214494479963,-4.97337279470518,-4.49935967199326));
#32510=CARTESIAN_POINT('Ctrl Pts',(9.97229944890177,-5.50399269762474,-3.78583316881013));
#32511=CARTESIAN_POINT('Ctrl Pts',(9.72884798379595,-5.74433681300753,-3.39271619660671));
#32512=CARTESIAN_POINT('Ctrl Pts',(9.31382031628678,-6.15730438613379,-2.51609523661562));
#32513=CARTESIAN_POINT('Ctrl Pts',(9.14962517763389,-6.32266022732949,-2.04686959132891));
#32514=CARTESIAN_POINT('Ctrl Pts',(8.97968417042009,-6.49418647715621,-1.29879006759369));
#32515=CARTESIAN_POINT('Ctrl Pts',(8.93575384240423,-6.53864733931865,-1.04005934340375));
#32516=CARTESIAN_POINT('Ctrl Pts',(8.87777246418902,-6.59736187089493,-0.523086822034743));
#32517=CARTESIAN_POINT('Ctrl Pts',(8.8631452526061,-6.61219755450612,-0.263005427051395));
#32518=CARTESIAN_POINT('Ctrl Pts',(8.86304815521195,-6.6122959841467,0.260400685698262));
#32519=CARTESIAN_POINT('Ctrl Pts',(8.87795718231789,-6.59717455971195,0.525795200917309));
#32520=CARTESIAN_POINT('Ctrl Pts',(8.93628291242789,-6.53811183992734,1.04370213362036));
#32521=CARTESIAN_POINT('Ctrl Pts',(8.97946099290913,-6.49441229642004,1.29752474849125));
#32522=CARTESIAN_POINT('Ctrl Pts',(9.09245107359478,-6.38036710627489,1.79547047261785));
#32523=CARTESIAN_POINT('Ctrl Pts',(9.16291409861826,-6.3093667473441,2.0412446593706));
#32524=CARTESIAN_POINT('Ctrl Pts',(9.32652223254246,-6.14517355622585,2.51312695721537));
#32525=CARTESIAN_POINT('Ctrl Pts',(9.41946362141348,-6.05218100166854,2.73949361055882));
#32526=CARTESIAN_POINT('Ctrl Pts',(9.62584947135055,-5.84682859048649,3.17490081246898));
#32527=CARTESIAN_POINT('Ctrl Pts',(9.73996892072135,-5.73380090596656,3.38497438741758));
#32528=CARTESIAN_POINT('Ctrl Pts',(9.98471062769431,-5.49326410523417,3.78353127448484));
#32529=CARTESIAN_POINT('Ctrl Pts',(10.1146920373345,-5.36637373914797,3.97129991678004));
#32530=CARTESIAN_POINT('Ctrl Pts',(10.5258167104531,-4.96921689661331,4.50410582808353));
#32531=CARTESIAN_POINT('Ctrl Pts',(10.828058423632,-4.68196521947166,4.81930905446431));
#32532=CARTESIAN_POINT('Ctrl Pts',(11.1585526803519,-4.38134327770267,5.09856534401067));
#32533=CARTESIAN_POINT('Origin',(14.8870768733179,0.,0.));
#32534=CARTESIAN_POINT('',(18.7837086993174,-4.27128032554705,-5.09745204146194));
#32535=CARTESIAN_POINT('Origin',(14.8870768733179,0.,-5.09745204146194));
#32536=CARTESIAN_POINT('',(14.8870768733179,-4.27128032554705,-6.41621047834285));
#32537=CARTESIAN_POINT('Origin',(14.8870768733179,-4.27128032554705,0.));
#32538=CARTESIAN_POINT('',(14.8870768733179,-4.71972237234598E-16,-7.70789157434132));
#32539=CARTESIAN_POINT('Origin',(14.8870768733179,0.,0.));
#32540=CARTESIAN_POINT('Origin',(14.8870768733179,-4.27128032554705,0.));
#32541=CARTESIAN_POINT('',(14.8870768733179,-4.71972237234598E-16,7.70789157434132));
#32542=CARTESIAN_POINT('Origin',(14.8870768733179,0.,0.));
#32543=CARTESIAN_POINT('Origin',(14.8870768733179,0.,5.09745204146194));
#32544=CARTESIAN_POINT('Origin',(-3.88784034431744,6.,0.));
#32545=CARTESIAN_POINT('Origin',(18.3575990203927,-10.,4.26678755349543));
#32546=CARTESIAN_POINT('',(18.4538614420533,0.,4.26678755349543));
#32547=CARTESIAN_POINT('',(18.3575990203927,0.,4.26678755349543));
#32548=CARTESIAN_POINT('',(18.7133976597241,-3.81977834524697,4.26678755349543));
#32549=CARTESIAN_POINT('Ctrl Pts',(18.4538614420644,-2.56528132069889E-12,
4.26678755349543));
#32550=CARTESIAN_POINT('Ctrl Pts',(18.4538614420546,-0.0764186347087233,
4.26678755349543));
#32551=CARTESIAN_POINT('Ctrl Pts',(18.4647576002876,-0.151683565594343,
4.266787553495));
#32552=CARTESIAN_POINT('Ctrl Pts',(18.4806164604976,-0.225114443517557,
4.26678755349578));
#32553=CARTESIAN_POINT('Ctrl Pts',(18.4822477496512,-0.232667760282275,
4.26678755349586));
#32554=CARTESIAN_POINT('Ctrl Pts',(18.4839315235274,-0.240201701574996,
4.26678755349596));
#32555=CARTESIAN_POINT('Ctrl Pts',(18.4856613288592,-0.247715549624222,
4.26678755349611));
#32556=CARTESIAN_POINT('Ctrl Pts',(18.4856957875747,-0.247865229791915,
4.26678755349611));
#32557=CARTESIAN_POINT('Ctrl Pts',(18.4857302630303,-0.248014904556736,
4.26678755349611));
#32558=CARTESIAN_POINT('Ctrl Pts',(18.4857647552007,-0.248164573924098,
4.26678755349611));
#32559=CARTESIAN_POINT('Ctrl Pts',(18.5043314682965,-0.32872976226667,4.26678755349766));
#32560=CARTESIAN_POINT('Ctrl Pts',(18.5277911787412,-0.407964970138364,
4.2667875534948));
#32561=CARTESIAN_POINT('Ctrl Pts',(18.552314823445,-0.486910969870589,4.26678755349595));
#32562=CARTESIAN_POINT('Ctrl Pts',(18.552357345021,-0.487047854430916,4.26678755349595));
#32563=CARTESIAN_POINT('Ctrl Pts',(18.55239986991,-0.487184738089763,4.26678755349595));
#32564=CARTESIAN_POINT('Ctrl Pts',(18.5524423981078,-0.487321620848336,
4.26678755349595));
#32565=CARTESIAN_POINT('Ctrl Pts',(18.6015459292246,-0.645367979461387,
4.26678755349831));
#32566=CARTESIAN_POINT('Ctrl Pts',(18.655043587707,-0.802219259702535,4.2667875534954));
#32567=CARTESIAN_POINT('Ctrl Pts',(18.7060174878535,-0.959758075388361,
4.26678755349545));
#32568=CARTESIAN_POINT('Ctrl Pts',(18.7060553290986,-0.959875026708893,
4.26678755349545));
#32569=CARTESIAN_POINT('Ctrl Pts',(18.7060931692692,-0.959991978323139,
4.26678755349545));
#32570=CARTESIAN_POINT('Ctrl Pts',(18.7061310083643,-0.960108930231384,
4.26678755349545));
#32571=CARTESIAN_POINT('Ctrl Pts',(18.8081234684985,-1.27534408100678,4.26678755349557));
#32572=CARTESIAN_POINT('Ctrl Pts',(18.9022854709063,-1.59271847963817,4.26678755349544));
#32573=CARTESIAN_POINT('Ctrl Pts',(18.9681979440421,-1.91781921667449,4.26678755349543));
#32574=CARTESIAN_POINT('Ctrl Pts',(18.9682142463112,-1.91789962451603,4.26678755349543));
#32575=CARTESIAN_POINT('Ctrl Pts',(18.968230546818,-1.91798003264918,4.26678755349543));
#32576=CARTESIAN_POINT('Ctrl Pts',(18.9682468455622,-1.91806044107386,4.26678755349543));
#32577=CARTESIAN_POINT('Ctrl Pts',(19.0011918379723,-2.08059167162913,4.26678755349543));
#32578=CARTESIAN_POINT('Ctrl Pts',(19.0269345328965,-2.24431257125727,4.26678755349543));
#32579=CARTESIAN_POINT('Ctrl Pts',(19.0420990825219,-2.40836704229758,4.26678755349543));
#32580=CARTESIAN_POINT('Ctrl Pts',(19.0572711744983,-2.57250310866618,4.26678755349543));
#32581=CARTESIAN_POINT('Ctrl Pts',(19.0621241707402,-2.73728491562089,4.26678755349543));
#32582=CARTESIAN_POINT('Ctrl Pts',(19.0510253633269,-2.90306553275185,4.26678755349543));
#32583=CARTESIAN_POINT('Ctrl Pts',(19.0510226192503,-2.90310652046414,4.26678755349543));
#32584=CARTESIAN_POINT('Ctrl Pts',(19.0510198741666,-2.90314750825434,4.26678755349543));
#32585=CARTESIAN_POINT('Ctrl Pts',(19.0510171280758,-2.9031884961222,4.26678755349543));
#32586=CARTESIAN_POINT('Ctrl Pts',(19.0454664098095,-2.98603794451841,4.26678755349543));
#32587=CARTESIAN_POINT('Ctrl Pts',(19.0358009037468,-3.06920490198507,4.26678755349543));
#32588=CARTESIAN_POINT('Ctrl Pts',(19.0211988493128,-3.15074112916623,4.26678755349543));
#32589=CARTESIAN_POINT('Ctrl Pts',(19.006589543518,-3.23231784712912,4.26678755349543));
#32590=CARTESIAN_POINT('Ctrl Pts',(18.9870649540648,-3.31269840555977,4.26678755349543));
#32591=CARTESIAN_POINT('Ctrl Pts',(18.9610497328516,-3.39149913067213,4.26678755349543));
#32592=CARTESIAN_POINT('Ctrl Pts',(18.9610433008161,-3.39151861346081,4.26678755349543));
#32593=CARTESIAN_POINT('Ctrl Pts',(18.9610368683589,-3.39153809619381,4.26678755349543));
#32594=CARTESIAN_POINT('Ctrl Pts',(18.9610304354799,-3.39155757887106,4.26678755349543));
#32595=CARTESIAN_POINT('Ctrl Pts',(18.9350182596588,-3.47033829694986,4.26678755349543));
#32596=CARTESIAN_POINT('Ctrl Pts',(18.9021092263951,-3.54820850188026,4.26678755349543));
#32597=CARTESIAN_POINT('Ctrl Pts',(18.8615965006036,-3.62042627660495,4.26678755349543));
#32598=CARTESIAN_POINT('Ctrl Pts',(18.861591491163,-3.62043520640779,4.26678755349543));
#32599=CARTESIAN_POINT('Ctrl Pts',(18.8615864816075,-3.6204441361364,4.26678755349543));
#32600=CARTESIAN_POINT('Ctrl Pts',(18.8615814719371,-3.62045306579077,4.26678755349543));
#32601=CARTESIAN_POINT('Ctrl Pts',(18.8293282449153,-3.67794390791935,4.26678755349543));
#32602=CARTESIAN_POINT('Ctrl Pts',(18.7923266345213,-3.73234026194883,4.26678755349543));
#32603=CARTESIAN_POINT('Ctrl Pts',(18.7484881342047,-3.78228112582125,4.26678755349543));
#32604=CARTESIAN_POINT('Ctrl Pts',(18.7372525105736,-3.79508075961879,4.26678755349543));
#32605=CARTESIAN_POINT('Ctrl Pts',(18.7255675768418,-3.8075875837349,4.26678755349543));
#32606=CARTESIAN_POINT('Ctrl Pts',(18.7133976597241,-3.81977834524697,4.26678755349543));
#32607=CARTESIAN_POINT('Origin',(14.8870768733179,0.,4.26678755349543));
#32608=CARTESIAN_POINT('Origin',(18.3575990203927,-10.,-4.26678755349543));
#32609=CARTESIAN_POINT('',(18.3843475112712,-4.12317055822481,-4.26678755349543));
#32610=CARTESIAN_POINT('Ctrl Pts',(18.3575990203927,-3.99420842564088,-4.26678755349543));
#32611=CARTESIAN_POINT('Ctrl Pts',(18.3575990203927,-4.03574406331344,-4.26678755349543));
#32612=CARTESIAN_POINT('Ctrl Pts',(18.3672627745756,-4.08260100655593,-4.26678755349543));
#32613=CARTESIAN_POINT('Ctrl Pts',(18.3843475112712,-4.1231705582248,-4.26678755349543));
#32614=CARTESIAN_POINT('',(18.7133976597241,-3.81977834524697,-4.26678755349543));
#32615=CARTESIAN_POINT('Origin',(14.8870768733179,0.,-4.26678755349543));
#32616=CARTESIAN_POINT('',(18.4538614420533,0.,-4.26678755349543));
#32617=CARTESIAN_POINT('Ctrl Pts',(18.7133976597241,-3.81977834524697,-4.26678755349543));
#32618=CARTESIAN_POINT('Ctrl Pts',(18.7608818058108,-3.77221286924961,-4.26678755349543));
#32619=CARTESIAN_POINT('Ctrl Pts',(18.8009866046437,-3.71983834098458,-4.26678755349543));
#32620=CARTESIAN_POINT('Ctrl Pts',(18.8358117274585,-3.66402313169491,-4.26678755349543));
#32621=CARTESIAN_POINT('Ctrl Pts',(18.8447418174152,-3.64971062395264,-4.26678755349543));
#32622=CARTESIAN_POINT('Ctrl Pts',(18.8533245106631,-3.63517172105021,-4.26678755349543));
#32623=CARTESIAN_POINT('Ctrl Pts',(18.8615948019429,-3.62042922728382,-4.26678755349543));
#32624=CARTESIAN_POINT('Ctrl Pts',(18.8615953571645,-3.62042823755431,-4.26678755349543));
#32625=CARTESIAN_POINT('Ctrl Pts',(18.8615959123847,-3.6204272478239,-4.26678755349543));
#32626=CARTESIAN_POINT('Ctrl Pts',(18.8615964676035,-3.62042625809258,-4.26678755349543));
#32627=CARTESIAN_POINT('Ctrl Pts',(18.9021180702506,-3.54819257345561,-4.26678755349543));
#32628=CARTESIAN_POINT('Ctrl Pts',(18.9350325943709,-3.4703043534866,-4.26678755349543));
#32629=CARTESIAN_POINT('Ctrl Pts',(18.9610475717044,-3.39150560137125,-4.26678755349543));
#32630=CARTESIAN_POINT('Ctrl Pts',(18.9610482846085,-3.39150344200163,-4.26678755349543));
#32631=CARTESIAN_POINT('Ctrl Pts',(18.9610489975074,-3.39150128263133,-4.26678755349543));
#32632=CARTESIAN_POINT('Ctrl Pts',(18.9610497104011,-3.39149912326034,-4.26678755349543));
#32633=CARTESIAN_POINT('Ctrl Pts',(18.9870650252034,-3.3126981536433,-4.26678755349543));
#32634=CARTESIAN_POINT('Ctrl Pts',(19.0065895569739,-3.23231768034818,-4.26678755349543));
#32635=CARTESIAN_POINT('Ctrl Pts',(19.0211988282645,-3.15074112539677,-4.26678755349543));
#32636=CARTESIAN_POINT('Ctrl Pts',(19.0358072958342,-3.06916905833388,-4.26678755349543));
#32637=CARTESIAN_POINT('Ctrl Pts',(19.0454748719371,-2.98596489662045,-4.26678755349543));
#32638=CARTESIAN_POINT('Ctrl Pts',(19.0510244255707,-2.90307915963347,-4.26678755349543));
#32639=CARTESIAN_POINT('Ctrl Pts',(19.0510247297345,-2.90307461677399,-4.26678755349543));
#32640=CARTESIAN_POINT('Ctrl Pts',(19.0510250338859,-2.90307007391548,-4.26678755349543));
#32641=CARTESIAN_POINT('Ctrl Pts',(19.051025338025,-2.90306553105792,-4.26678755349543));
#32642=CARTESIAN_POINT('Ctrl Pts',(19.062124153563,-2.73728499936675,-4.26678755349543));
#32643=CARTESIAN_POINT('Ctrl Pts',(19.0572711633294,-2.57250305359533,-4.26678755349543));
#32644=CARTESIAN_POINT('Ctrl Pts',(19.0420990719329,-2.40836704327638,-4.26678755349543));
#32645=CARTESIAN_POINT('Ctrl Pts',(19.0269278165402,-2.24424007708595,-4.26678755349543));
#32646=CARTESIAN_POINT('Ctrl Pts',(19.0011690644904,-2.08044717424057,-4.26678755349543));
#32647=CARTESIAN_POINT('Ctrl Pts',(18.9682033134569,-1.91784596289597,-4.26678755349543));
#32648=CARTESIAN_POINT('Ctrl Pts',(18.9682015066474,-1.91783705093721,-4.26678755349543));
#32649=CARTESIAN_POINT('Ctrl Pts',(18.9681996998163,-1.91782813898203,-4.26678755349543));
#32650=CARTESIAN_POINT('Ctrl Pts',(18.9681978929635,-1.91781922703043,-4.26678755349543));
#32651=CARTESIAN_POINT('Ctrl Pts',(18.9022638977272,-1.59261256156863,-4.26678755349543));
#32652=CARTESIAN_POINT('Ctrl Pts',(18.8080608958824,-1.27513481155645,-4.26678755349543));
#32653=CARTESIAN_POINT('Ctrl Pts',(18.7060299372189,-0.959797005169111,
-4.26678755349543));
#32654=CARTESIAN_POINT('Ctrl Pts',(18.7060257431389,-0.959784042907454,
-4.26678755349543));
#32655=CARTESIAN_POINT('Ctrl Pts',(18.7060215490457,-0.95977108064926,-4.26678755349543));
#32656=CARTESIAN_POINT('Ctrl Pts',(18.7060173549391,-0.959758118394527,
-4.26678755349543));
#32657=CARTESIAN_POINT('Ctrl Pts',(18.6550043488165,-0.802097940920412,
-4.26678755349543));
#32658=CARTESIAN_POINT('Ctrl Pts',(18.6014547932599,-0.64510416345673,-4.26678755349549));
#32659=CARTESIAN_POINT('Ctrl Pts',(18.5523323438895,-0.486969437517935,
-4.26678755349544));
#32660=CARTESIAN_POINT('Ctrl Pts',(18.5523263086478,-0.486950008900037,
-4.26678755349544));
#32661=CARTESIAN_POINT('Ctrl Pts',(18.552320273473,-0.486930580264954,-4.26678755349544));
#32662=CARTESIAN_POINT('Ctrl Pts',(18.552314238365,-0.486911151612686,-4.26678755349544));
#32663=CARTESIAN_POINT('Ctrl Pts',(18.5277575741225,-0.40785657677535,-4.26678755349541));
#32664=CARTESIAN_POINT('Ctrl Pts',(18.5042740984017,-0.328527131581695,
-4.266787553496));
#32665=CARTESIAN_POINT('Ctrl Pts',(18.4857119715276,-0.247937289204806,
-4.2667875534956));
#32666=CARTESIAN_POINT('Ctrl Pts',(18.4856949543482,-0.247863406948809,
-4.2667875534956));
#32667=CARTESIAN_POINT('Ctrl Pts',(18.4856779414224,-0.247789524151342,
-4.2667875534956));
#32668=CARTESIAN_POINT('Ctrl Pts',(18.4856609327526,-0.247715640809645,
-4.2667875534956));
#32669=CARTESIAN_POINT('Ctrl Pts',(18.4781251595079,-0.214981269683404,
-4.26678755349544));
#32670=CARTESIAN_POINT('Ctrl Pts',(18.4714946508473,-0.182018340757567,
-4.26678755349544));
#32671=CARTESIAN_POINT('Ctrl Pts',(18.4662508311777,-0.148698263420427,
-4.26678755349543));
#32672=CARTESIAN_POINT('Ctrl Pts',(18.4619453320882,-0.121340426637857,
-4.26678755349543));
#32673=CARTESIAN_POINT('Ctrl Pts',(18.4585740060291,-0.0937414373303757,
-4.26678755349543));
#32674=CARTESIAN_POINT('Ctrl Pts',(18.4564380870412,-0.0658241261208444,
-4.26678755349543));
#32675=CARTESIAN_POINT('Ctrl Pts',(18.4547751193048,-0.0440884759903845,
-4.26678755349543));
#32676=CARTESIAN_POINT('Ctrl Pts',(18.4538614420616,-0.0221597443920782,
-4.26678755349543));
#32677=CARTESIAN_POINT('Ctrl Pts',(18.4538614420644,-2.56805687826045E-12,
-4.26678755349543));
#32678=CARTESIAN_POINT('',(18.3575990203927,0.,-4.26678755349543));
#32679=CARTESIAN_POINT('Origin',(14.8870768733179,0.,0.));
#32680=CARTESIAN_POINT('Origin',(18.4538614420533,1.29836352043984E-18,
-4.76678755349543));
#32681=CARTESIAN_POINT('Origin',(14.8870768733179,0.,0.));
#32682=CARTESIAN_POINT('Origin',(18.4538614420533,3.76800988090885E-16,
4.76678755349543));
#32683=CARTESIAN_POINT('Ctrl Pts',(18.6542359870042,-4.26970425052901,-5.14005510487642));
#32684=CARTESIAN_POINT('Ctrl Pts',(19.0577899084937,-5.18691783079565,-4.26678755349586));
#32685=CARTESIAN_POINT('Ctrl Pts',(18.5204132448321,-3.96090161554629,-4.26678755349543));
#32686=CARTESIAN_POINT('Ctrl Pts',(18.9222117185918,-4.16007568622317,-5.11560140424043));
#32687=CARTESIAN_POINT('Ctrl Pts',(19.4799272843404,-4.78635337341915,-4.26678755349528));
#32688=CARTESIAN_POINT('Ctrl Pts',(18.6801136214415,-3.87779830058524,-4.26678755349543));
#32689=CARTESIAN_POINT('Ctrl Pts',(19.0979593370657,-4.00248991871804,-5.07972521647459));
#32690=CARTESIAN_POINT('Ctrl Pts',(19.6110505295027,-4.40503233983348,-4.26678755349543));
#32691=CARTESIAN_POINT('Ctrl Pts',(18.7844712393506,-3.75790943902247,-4.26678755349543));
#32692=CARTESIAN_POINT('Ctrl Pts',(19.2959765085615,-3.73301197651848,-5.01655082533848));
#32693=CARTESIAN_POINT('Ctrl Pts',(19.68659106153,-3.91712710693031,-4.26678755349543));
#32694=CARTESIAN_POINT('Ctrl Pts',(18.9021191809457,-3.54819059360291,-4.26678755349543));
#32695=CARTESIAN_POINT('Ctrl Pts',(19.3513956440603,-3.63388752247013,-4.99301158143074));
#32696=CARTESIAN_POINT('Ctrl Pts',(19.6930611405989,-3.7699368058973,-4.26678755349543));
#32697=CARTESIAN_POINT('Ctrl Pts',(18.9350343692454,-3.47030011905697,-4.26678755349543));
#32698=CARTESIAN_POINT('Ctrl Pts',(19.4390223899416,-3.43576678210827,-4.94534871538099));
#32699=CARTESIAN_POINT('Ctrl Pts',(19.6880690365751,-3.50527002686798,-4.26678755349543));
#32700=CARTESIAN_POINT('Ctrl Pts',(18.9870650305019,-3.31269812051263,-4.26678755349543));
#32701=CARTESIAN_POINT('Ctrl Pts',(19.4719166463349,-3.33589127417514,-4.92102514232829));
#32702=CARTESIAN_POINT('Ctrl Pts',(19.6779161308525,-3.38370254509204,-4.26678755349543));
#32703=CARTESIAN_POINT('Ctrl Pts',(19.0065895537831,-3.23231765789036,-4.26678755349543));
#32704=CARTESIAN_POINT('Ctrl Pts',(19.5211651350852,-3.13583705072043,-4.87181032321129));
#32705=CARTESIAN_POINT('Ctrl Pts',(19.6488720310131,-3.15520989470188,-4.26678755349543));
#32706=CARTESIAN_POINT('Ctrl Pts',(19.0358080846578,-3.06916458966381,-4.26678755349543));
#32707=CARTESIAN_POINT('Ctrl Pts',(19.5374740961704,-3.03514253616215,-4.84678973600571));
#32708=CARTESIAN_POINT('Ctrl Pts',(19.6302244752384,-3.04627737812982,-4.26678755349543));
#32709=CARTESIAN_POINT('Ctrl Pts',(19.0454759169275,-2.98595579110855,-4.26678755349543));
#32710=CARTESIAN_POINT('Ctrl Pts',(19.5656064151764,-2.73847376165093,-4.77259844285197));
#32711=CARTESIAN_POINT('Ctrl Pts',(19.5684120549786,-2.74532693995999,-4.26678755349543));
#32712=CARTESIAN_POINT('Ctrl Pts',(19.0621241480217,-2.73728500880102,-4.26678755349543));
#32713=CARTESIAN_POINT('Ctrl Pts',(19.557505688877,-2.54754173168078,-4.72420514209177));
#32714=CARTESIAN_POINT('Ctrl Pts',(19.5170237058281,-2.55560043450117,-4.26678755349543));
#32715=CARTESIAN_POINT('Ctrl Pts',(19.057271160227,-2.57250304610011,-4.26678755349543));
#32716=CARTESIAN_POINT('Ctrl Pts',(19.5065540718371,-2.17859460722192,-4.63142824827105));
#32717=CARTESIAN_POINT('Ctrl Pts',(19.4034908984912,-2.19830057322816,-4.26678755349543));
#32718=CARTESIAN_POINT('Ctrl Pts',(19.0269269806048,-2.2442310407331,-4.26678755349543));
#32719=CARTESIAN_POINT('Ctrl Pts',(19.463245787281,-2.00027050534638,-4.58697424177898));
#32720=CARTESIAN_POINT('Ctrl Pts',(19.3409663838283,-2.02616314418212,-4.26678755349543));
#32721=CARTESIAN_POINT('Ctrl Pts',(19.0011662279257,-2.08042916291789,-4.26678755349543));
#32722=CARTESIAN_POINT('Ctrl Pts',(19.2968891634531,-1.48548484252353,-4.46363148732574));
#32723=CARTESIAN_POINT('Ctrl Pts',(19.1483011492445,-1.54320588831284,-4.26678755349543));
#32724=CARTESIAN_POINT('Ctrl Pts',(18.9022612159307,-1.59259935669665,-4.26678755349543));
#32725=CARTESIAN_POINT('Ctrl Pts',(19.1383625511518,-1.17253950176775,-4.39559658478723));
#32726=CARTESIAN_POINT('Ctrl Pts',(18.9990590372986,-1.2248828326142,-4.26678755349543));
#32727=CARTESIAN_POINT('Ctrl Pts',(18.8080530853766,-1.27510872906601,-4.26678755349543));
#32728=CARTESIAN_POINT('Ctrl Pts',(18.8807693660449,-0.726865400089183,
-4.32494765329133));
#32729=CARTESIAN_POINT('Ctrl Pts',(18.7752223218753,-0.764223859480729,
-4.26678755349543));
#32730=CARTESIAN_POINT('Ctrl Pts',(18.6549994601397,-0.802082822630004,
-4.26678755349543));
#32731=CARTESIAN_POINT('Ctrl Pts',(18.7906375006256,-0.582332400014721,
-4.30661231556638));
#32732=CARTESIAN_POINT('Ctrl Pts',(18.70016617769,-0.613489035379009,-4.26678755349543));
#32733=CARTESIAN_POINT('Ctrl Pts',(18.6014509972619,-0.645096921999166,
-4.26678755349543));
#32734=CARTESIAN_POINT('Ctrl Pts',(18.6665728209963,-0.366692065764295,
-4.28782126317335));
#32735=CARTESIAN_POINT('Ctrl Pts',(18.5987003778136,-0.387079548706928,
-4.26678755349543));
#32736=CARTESIAN_POINT('Ctrl Pts',(18.5277457016063,-0.407818315284394,
-4.26678755349543));
#32737=CARTESIAN_POINT('Ctrl Pts',(18.6270102662637,-0.295011052175803,
-4.28300214458113));
#32738=CARTESIAN_POINT('Ctrl Pts',(18.5666581019247,-0.31158967965086,-4.26678755349536));
#32739=CARTESIAN_POINT('Ctrl Pts',(18.5042426057229,-0.328435858715435,
-4.26678755349543));
#32740=CARTESIAN_POINT('Ctrl Pts',(18.5361976874514,-0.0841343764222963,
-4.27345035595134));
#32741=CARTESIAN_POINT('Ctrl Pts',(18.4936062418503,-0.0895865205474039,
-4.26678755349556));
#32742=CARTESIAN_POINT('Ctrl Pts',(18.4502940130769,-0.0940844251823421,
-4.26678755349543));
#32743=CARTESIAN_POINT('Ctrl Pts',(18.5093786690843,0.0599803308146132,
-4.27270022961939));
#32744=CARTESIAN_POINT('Ctrl Pts',(18.4720206072776,0.0639366199169896,
-4.26678755349649));
#32745=CARTESIAN_POINT('Ctrl Pts',(18.4343618285263,0.0671004789595955,
-4.26678755349543));
#32746=CARTESIAN_POINT('Ctrl Pts',(18.6063997166192,0.207276912386747,-4.27916424911031));
#32747=CARTESIAN_POINT('Ctrl Pts',(18.5500685617386,0.219135615093589,-4.26678755349219));
#32748=CARTESIAN_POINT('Ctrl Pts',(18.4919985205465,0.231010279447602,-4.26678755349543));
#32749=CARTESIAN_POINT('Origin',(18.7133976597241,-3.81977834524697,-4.76678755349543));
#32750=CARTESIAN_POINT('Origin',(14.8870768733179,0.,-4.76678755349543));
#32751=CARTESIAN_POINT('Ctrl Pts',(18.7837086993174,-4.27128032554705,-5.09745204146194));
#32752=CARTESIAN_POINT('Ctrl Pts',(18.7837837624154,-4.27218856939587,-5.09663362133658));
#32753=CARTESIAN_POINT('Ctrl Pts',(18.7838569011206,-4.27309483878909,-5.0958128351685));
#32754=CARTESIAN_POINT('Ctrl Pts',(18.787810353939,-4.32329670754872,-5.05011558445576));
#32755=CARTESIAN_POINT('Ctrl Pts',(18.7859513395349,-4.36654052586954,-4.99838378394199));
#32756=CARTESIAN_POINT('Ctrl Pts',(18.7708050164925,-4.43566404078374,-4.88679567157663));
#32757=CARTESIAN_POINT('Ctrl Pts',(18.7578033695063,-4.46162539414925,-4.82752476395243));
#32758=CARTESIAN_POINT('Ctrl Pts',(18.7204855200627,-4.49373583225153,-4.70302915637018));
#32759=CARTESIAN_POINT('Ctrl Pts',(18.6958976213804,-4.49858998809844,-4.63853166786264));
#32760=CARTESIAN_POINT('Ctrl Pts',(18.6406738757079,-4.48244009347221,-4.52164441884446));
#32761=CARTESIAN_POINT('Ctrl Pts',(18.6114407022608,-4.46403154155928,-4.46994402103078));
#32762=CARTESIAN_POINT('Ctrl Pts',(18.5512951506147,-4.40736654541262,-4.38235276133824));
#32763=CARTESIAN_POINT('Ctrl Pts',(18.5214085776067,-4.37097137724525,-4.34705233647852));
#32764=CARTESIAN_POINT('Ctrl Pts',(18.4626511753395,-4.28318578164407,-4.29387508247684));
#32765=CARTESIAN_POINT('Ctrl Pts',(18.4346965748636,-4.2329044689914,-4.27709516144855));
#32766=CARTESIAN_POINT('Ctrl Pts',(18.4006544833022,-4.16080775958966,-4.26793451055797));
#32767=CARTESIAN_POINT('Ctrl Pts',(18.3923049583211,-4.14206637529222,-4.26678755349543));
#32768=CARTESIAN_POINT('Ctrl Pts',(18.3843475112712,-4.1231705582248,-4.26678755349543));
#32769=CARTESIAN_POINT('Origin',(14.8870768733179,-3.99420842564088,0.));
#32770=CARTESIAN_POINT('Ctrl Pts',(11.1585526803519,-4.38134327770264,-5.09856534401066));
#32771=CARTESIAN_POINT('Ctrl Pts',(11.1773095544415,-4.40043210711516,-5.08334924385387));
#32772=CARTESIAN_POINT('Ctrl Pts',(11.1965634146953,-4.41737314983265,-5.0663896003135));
#32773=CARTESIAN_POINT('Ctrl Pts',(11.2160327360732,-4.43193019040154,-5.04794583054052));
#32774=CARTESIAN_POINT('Ctrl Pts',(11.235499063637,-4.44648499252185,-5.02950489688177));
#32775=CARTESIAN_POINT('Ctrl Pts',(11.2551808637128,-4.45865655224405,-5.0095803001658));
#32776=CARTESIAN_POINT('Ctrl Pts',(11.2747924288633,-4.46825273215176,-4.98845874515855));
#32777=CARTESIAN_POINT('Ctrl Pts',(11.2941553527337,-4.47772724882462,-4.9676049755338));
#32778=CARTESIAN_POINT('Ctrl Pts',(11.3134499541213,-4.48469120824842,-4.94558445055882));
#32779=CARTESIAN_POINT('Ctrl Pts',(11.3323953866326,-4.48900270879227,-4.9226994094508));
#32780=CARTESIAN_POINT('Ctrl Pts',(11.3351876321147,-4.48963815313524,-4.91932653038861));
#32781=CARTESIAN_POINT('Ctrl Pts',(11.3379722800483,-4.4902160597842,-4.91593491878871));
#32782=CARTESIAN_POINT('Ctrl Pts',(11.3407484170919,-4.49073605743578,-4.91252559036193));
#32783=CARTESIAN_POINT('Ctrl Pts',(11.3547633161217,-4.49336118525482,-4.89531412244419));
#32784=CARTESIAN_POINT('Ctrl Pts',(11.3685552099567,-4.49450846568627,-4.87762256908707));
#32785=CARTESIAN_POINT('Ctrl Pts',(11.3819878602132,-4.49414152262891,-4.85965719763253));
#32786=CARTESIAN_POINT('Ctrl Pts',(11.3954056409517,-4.49377498576589,-4.84171171327456));
#32787=CARTESIAN_POINT('Ctrl Pts',(11.4084645659427,-4.49189752730234,-4.82349370723202));
#32788=CARTESIAN_POINT('Ctrl Pts',(11.4210277728046,-4.48852481095031,-4.80521097378418));
#32789=CARTESIAN_POINT('Ctrl Pts',(11.433582228137,-4.48515444403239,-4.78694097608782));
#32790=CARTESIAN_POINT('Ctrl Pts',(11.4456412560894,-4.48029104788819,-4.76860702043759));
#32791=CARTESIAN_POINT('Ctrl Pts',(11.4570732740616,-4.47400139883439,-4.75040836654757));
#32792=CARTESIAN_POINT('Ctrl Pts',(11.468515105606,-4.46770635056538,-4.73219409041087));
#32793=CARTESIAN_POINT('Ctrl Pts',(11.4793284781849,-4.4599829216249,-4.71411597746034));
#32794=CARTESIAN_POINT('Ctrl Pts',(11.4893922899614,-4.45094580241366,-4.69635581925028));
#32795=CARTESIAN_POINT('Ctrl Pts',(11.492098904207,-4.44851531224363,-4.69157930928745));
#32796=CARTESIAN_POINT('Ctrl Pts',(11.4947513791465,-4.44599005094159,-4.68682566810472));
#32797=CARTESIAN_POINT('Ctrl Pts',(11.4973475437834,-4.44337278306917,-4.68209812382677));
#32798=CARTESIAN_POINT('Ctrl Pts',(11.5077296350375,-4.43290629974145,-4.66319262168548));
#32799=CARTESIAN_POINT('Ctrl Pts',(11.5172734125901,-4.42090574709506,-4.64460238394084));
#32800=CARTESIAN_POINT('Ctrl Pts',(11.5258955869577,-4.407513147548,-4.62655201641156));
#32801=CARTESIAN_POINT('Ctrl Pts',(11.5345249584581,-4.39410936888171,-4.60848658181409));
#32802=CARTESIAN_POINT('Ctrl Pts',(11.542230869974,-4.37931167764791,-4.59096238287243));
#32803=CARTESIAN_POINT('Ctrl Pts',(11.5489433162915,-4.36330323603274,-4.57417465116145));
#32804=CARTESIAN_POINT('Ctrl Pts',(11.5556857006915,-4.34722339540373,-4.55731204473639));
#32805=CARTESIAN_POINT('Ctrl Pts',(11.5614254453184,-4.32992254541936,-4.54119286157343));
#32806=CARTESIAN_POINT('Ctrl Pts',(11.5661098411331,-4.31161973967097,-4.52597841654605));
#32807=CARTESIAN_POINT('Ctrl Pts',(11.5705971850957,-4.29408685216031,-4.51140397605482));
#32808=CARTESIAN_POINT('Ctrl Pts',(11.5741160472694,-4.27563526415019,-4.49765968024976));
#32809=CARTESIAN_POINT('Ctrl Pts',(11.5766390463655,-4.25647826147464,-4.48485227017963));
#32810=CARTESIAN_POINT('Ctrl Pts',(11.5794931650594,-4.23480708468317,-4.47036400953826));
#32811=CARTESIAN_POINT('Ctrl Pts',(11.5810960704834,-4.21214692058059,-4.45702539669295));
#32812=CARTESIAN_POINT('Ctrl Pts',(11.5814513272679,-4.18878092056111,-4.44498843496028));
#32813=CARTESIAN_POINT('Ctrl Pts',(11.5818079107881,-4.1653276582881,-4.4329065202016));
#32814=CARTESIAN_POINT('Ctrl Pts',(11.5809072717996,-4.14116392284387,-4.42213601636339));
#32815=CARTESIAN_POINT('Ctrl Pts',(11.5787776008217,-4.11659012936366,-4.41278615285239));
#32816=CARTESIAN_POINT('Ctrl Pts',(11.5766350578908,-4.09186780931835,-4.40337977779331));
#32817=CARTESIAN_POINT('Ctrl Pts',(11.5732483837194,-4.06673113284847,-4.39541118322439));
#32818=CARTESIAN_POINT('Ctrl Pts',(11.5686744386717,-4.04149025072602,-4.388947118107));
#32819=CARTESIAN_POINT('Ctrl Pts',(11.5658212792752,-4.02574536108437,-4.38491492971454));
#32820=CARTESIAN_POINT('Ctrl Pts',(11.5625067173491,-4.0099599694054,-4.38146728159009));
#32821=CARTESIAN_POINT('Ctrl Pts',(11.5587504889214,-3.99420842564088,-4.37861204937474));
#32822=CARTESIAN_POINT('Ctrl Pts',(11.6023844202601,-3.95458824321301,-4.41143916299716));
#32823=CARTESIAN_POINT('Ctrl Pts',(12.0832028940249,-4.85453203063264,-4.76944949788135));
#32824=CARTESIAN_POINT('Ctrl Pts',(11.2797574433457,-4.27163583400664,-5.19835981118057));
#32825=CARTESIAN_POINT('Ctrl Pts',(11.2965510773294,-4.23166746059414,-4.18372017236837));
#32826=CARTESIAN_POINT('Ctrl Pts',(11.7265205257192,-5.02989742734166,-4.55166507795904));
#32827=CARTESIAN_POINT('Ctrl Pts',(10.9461377790192,-4.57173371007227,-4.93102752573452));
#32828=CARTESIAN_POINT('Ctrl Pts',(11.0041813520405,-4.50935327267487,-3.91588406330021));
#32829=CARTESIAN_POINT('Ctrl Pts',(11.35463790312,-5.24827427945486,-4.26941570590351));
#32830=CARTESIAN_POINT('Ctrl Pts',(10.6271700716899,-4.8726684807913,-4.61619738710776));
#32831=CARTESIAN_POINT('Ctrl Pts',(10.4769208212593,-5.01960677357028,-3.31082304312022));
#32832=CARTESIAN_POINT('Ctrl Pts',(10.7063724913704,-5.66598932993541,-3.61715501248506));
#32833=CARTESIAN_POINT('Ctrl Pts',(10.0519760808134,-5.42585676036716,-3.90424156632786));
#32834=CARTESIAN_POINT('Ctrl Pts',(10.2416197998638,-5.25263344048483,-2.97536444930372));
#32835=CARTESIAN_POINT('Ctrl Pts',(10.4143336358881,-5.8700643207334,-3.25312151833443));
#32836=CARTESIAN_POINT('Ctrl Pts',(9.79528424049654,-5.67861782892684,-3.50918796214299));
#32837=CARTESIAN_POINT('Ctrl Pts',(9.93843086546135,-5.55540857377054,-2.40970308249717));
#32838=CARTESIAN_POINT('Ctrl Pts',(10.0432225556495,-6.13934804787589,-2.62610418078175));
#32839=CARTESIAN_POINT('Ctrl Pts',(9.46453287938951,-6.00714081830833,-2.8425598401767));
#32840=CARTESIAN_POINT('Ctrl Pts',(9.84630047984833,-5.64795878660729,-2.2110461725345));
#32841=CARTESIAN_POINT('Ctrl Pts',(9.93245569216299,-6.22144594389688,-2.40973271653319));
#32842=CARTESIAN_POINT('Ctrl Pts',(9.36402698495814,-6.10758192572937,-2.60837180214158));
#32843=CARTESIAN_POINT('Ctrl Pts',(9.68617352369147,-5.80932527533534,-1.80243062942356));
#32844=CARTESIAN_POINT('Ctrl Pts',(9.74203346991433,-6.36432738273618,-1.96549235930559));
#32845=CARTESIAN_POINT('Ctrl Pts',(9.18934290808578,-6.28272973353952,-2.1265495309748));
#32846=CARTESIAN_POINT('Ctrl Pts',(9.61741694726934,-5.8789033577973,-1.59116370555004));
#32847=CARTESIAN_POINT('Ctrl Pts',(9.65983154833276,-6.42693601101231,-1.73484105847517));
#32848=CARTESIAN_POINT('Ctrl Pts',(9.11433573142727,-6.35826284245593,-1.87737372989252));
#32849=CARTESIAN_POINT('Ctrl Pts',(9.50459929783986,-5.99327376404412,-1.15327916114787));
#32850=CARTESIAN_POINT('Ctrl Pts',(9.52636981824612,-6.52928853743275,-1.25828708926425));
#32851=CARTESIAN_POINT('Ctrl Pts',(8.99126185288356,-6.48243255916743,-1.36082662439774));
#32852=CARTESIAN_POINT('Ctrl Pts',(9.4604583322397,-6.03814934571557,-0.924683260137496));
#32853=CARTESIAN_POINT('Ctrl Pts',(9.47377323241263,-6.57003899685759,-1.00827566940964));
#32854=CARTESIAN_POINT('Ctrl Pts',(8.94310807720623,-6.53115944545418,-1.0911207364409));
#32855=CARTESIAN_POINT('Ctrl Pts',(9.40208193744606,-6.09753305073092,-0.466967317285123));
#32856=CARTESIAN_POINT('Ctrl Pts',(9.40492964574317,-6.6235022859682,-0.509879942965713));
#32857=CARTESIAN_POINT('Ctrl Pts',(8.87942469755632,-6.59564165953961,-0.551041961059405));
#32858=CARTESIAN_POINT('Ctrl Pts',(9.3872659867011,-6.1126296856763,-0.236515666537748));
#32859=CARTESIAN_POINT('Ctrl Pts',(9.38729967348299,-6.63727567478022,-0.257585124159667));
#32860=CARTESIAN_POINT('Ctrl Pts',(8.86326184534119,-6.61203578049681,-0.279099068085999));
#32861=CARTESIAN_POINT('Ctrl Pts',(9.38689134318635,-6.11301121950842,0.22763695481613));
#32862=CARTESIAN_POINT('Ctrl Pts',(9.38685830965689,-6.63761983283789,0.247898500448822));
#32863=CARTESIAN_POINT('Ctrl Pts',(8.86285314380986,-6.61245009557666,0.268621792442221));
#32864=CARTESIAN_POINT('Ctrl Pts',(9.40176342855522,-6.09785739024047,0.463304811352815));
#32865=CARTESIAN_POINT('Ctrl Pts',(9.40455284931414,-6.62379599714687,0.505887165407633));
#32866=CARTESIAN_POINT('Ctrl Pts',(8.87907723400249,-6.59599386455161,0.546720178855904));
#32867=CARTESIAN_POINT('Ctrl Pts',(9.4598972513562,-6.03871977872338,0.921431650466073));
#32868=CARTESIAN_POINT('Ctrl Pts',(9.47310966312735,-6.57055322886647,1.00473113009131));
#32869=CARTESIAN_POINT('Ctrl Pts',(8.94249598790001,-6.53177883552457,1.08728425276695));
#32870=CARTESIAN_POINT('Ctrl Pts',(9.50290925766476,-5.99499017867409,1.14539763783599));
#32871=CARTESIAN_POINT('Ctrl Pts',(9.52436700384407,-6.53083458388161,1.24969833999858));
#32872=CARTESIAN_POINT('Ctrl Pts',(8.98941817134168,-6.48429618975125,1.35152822695961));
#32873=CARTESIAN_POINT('Ctrl Pts',(9.61518610363573,-5.88116189868735,1.58378166890141));
#32874=CARTESIAN_POINT('Ctrl Pts',(9.65718258741704,-6.42895757477472,1.72680004328843));
#32875=CARTESIAN_POINT('Ctrl Pts',(9.11190208330511,-6.36071474771872,1.86866655378836));
#32876=CARTESIAN_POINT('Ctrl Pts',(9.68512122038265,-5.81038739427925,1.7995430161374));
#32877=CARTESIAN_POINT('Ctrl Pts',(9.74079777647695,-6.36525992343917,1.96238829694538));
#32878=CARTESIAN_POINT('Ctrl Pts',(9.18819493952837,-6.28388263584057,2.12314424680613));
#32879=CARTESIAN_POINT('Ctrl Pts',(9.84601632803572,-5.64824348202644,2.21052171688795));
#32880=CARTESIAN_POINT('Ctrl Pts',(9.93213061479567,-6.2216843877734,2.40920076822843));
#32881=CARTESIAN_POINT('Ctrl Pts',(9.36371699951435,-6.10789086343246,2.60775370952373));
#32882=CARTESIAN_POINT('Ctrl Pts',(9.9370833975153,-5.55676033002984,2.40689371529671));
#32883=CARTESIAN_POINT('Ctrl Pts',(10.0415975635527,-6.14054654730368,2.62303197976634));
#32884=CARTESIAN_POINT('Ctrl Pts',(9.46306291377357,-6.00860775242521,2.83924822810719));
#32885=CARTESIAN_POINT('Ctrl Pts',(10.1385376408381,-5.35556888418775,2.78333395855106));
#32886=CARTESIAN_POINT('Ctrl Pts',(10.2829804663152,-5.96535627785836,3.03152616052292));
#32887=CARTESIAN_POINT('Ctrl Pts',(9.68283135755879,-5.79030632466165,3.28288272234244));
#32888=CARTESIAN_POINT('Ctrl Pts',(10.2496800262008,-5.24511502447779,2.96433987393686));
#32889=CARTESIAN_POINT('Ctrl Pts',(10.4176330616188,-5.86950598460442,3.22787521677906));
#32890=CARTESIAN_POINT('Ctrl Pts',(9.80407764728161,-5.67047963099968,3.49612647446564));
#32891=CARTESIAN_POINT('Ctrl Pts',(10.4853605723167,-5.01279790466392,3.30418734507658));
#32892=CARTESIAN_POINT('Ctrl Pts',(10.7029082049272,-5.67232521767017,3.59542004999764));
#32893=CARTESIAN_POINT('Ctrl Pts',(10.0611839441483,-5.41850504752442,3.89635328060898));
#32894=CARTESIAN_POINT('Ctrl Pts',(10.6100710485857,-4.89074738772537,3.46366781290886));
#32895=CARTESIAN_POINT('Ctrl Pts',(10.8555706827195,-5.56984011245734,3.76732714942));
#32896=CARTESIAN_POINT('Ctrl Pts',(10.1972318335047,-5.28615378358059,4.08409029398417));
#32897=CARTESIAN_POINT('Ctrl Pts',(11.0032082744194,-4.5103029492058,3.91467225682926));
#32898=CARTESIAN_POINT('Ctrl Pts',(11.3532021212208,-5.24922620608444,4.26785123513628));
#32899=CARTESIAN_POINT('Ctrl Pts',(10.6261085431467,-4.87369823287049,4.61477103735768));
#32900=CARTESIAN_POINT('Ctrl Pts',(11.2905193056397,-4.23711761886764,4.17928334636283));
#32901=CARTESIAN_POINT('Ctrl Pts',(11.7200923343516,-5.03301753809122,4.54780361973909));
#32902=CARTESIAN_POINT('Ctrl Pts',(10.9395311093629,-4.57766067780649,4.92579774106571));
#32903=CARTESIAN_POINT('Ctrl Pts',(11.6028786121923,-3.95414052617678,4.41180708798777));
#32904=CARTESIAN_POINT('Ctrl Pts',(12.0838277141608,-4.85422486814698,4.7698309482503));
#32905=CARTESIAN_POINT('Ctrl Pts',(11.2802965629704,-4.2711508971833,5.1987917615104));
#32906=CARTESIAN_POINT('Origin',(14.8870768733179,0.,4.76678755349543));
#32907=CARTESIAN_POINT('Origin',(18.7133976597241,-3.81977834524697,4.76678755349543));
#32908=CARTESIAN_POINT('Ctrl Pts',(18.3213959387515,-4.03643772855571,4.26678755349542));
#32909=CARTESIAN_POINT('Ctrl Pts',(18.3628668507259,-5.69599427429396,4.26678755349538));
#32910=CARTESIAN_POINT('Ctrl Pts',(18.3206061393696,-4.3689680817557,5.16231907827289));
#32911=CARTESIAN_POINT('Ctrl Pts',(18.6000581110489,-3.96321773775833,4.26678755349543));
#32912=CARTESIAN_POINT('Ctrl Pts',(19.3550672533386,-5.12141477481277,4.26678755349543));
#32913=CARTESIAN_POINT('Ctrl Pts',(18.7871890557531,-4.27257317214253,5.14144467458254));
#32914=CARTESIAN_POINT('Ctrl Pts',(18.7562374053204,-3.80823898150579,4.26678755349543));
#32915=CARTESIAN_POINT('Ctrl Pts',(19.5903948914683,-4.54592068587282,4.26678755349542));
#32916=CARTESIAN_POINT('Ctrl Pts',(19.0502150680539,-4.06694516153942,5.09523814558191));
#32917=CARTESIAN_POINT('Ctrl Pts',(18.9021191809457,-3.54819059360296,4.26678755349543));
#32918=CARTESIAN_POINT('Ctrl Pts',(19.6873927813158,-3.91750415511995,4.26678755349543));
#32919=CARTESIAN_POINT('Ctrl Pts',(19.2957763038374,-3.73291761076936,5.01693471360131));
#32920=CARTESIAN_POINT('Ctrl Pts',(18.9350343692453,-3.47030011905699,4.26678755349543));
#32921=CARTESIAN_POINT('Ctrl Pts',(19.6938018869037,-3.77022961187328,4.26678755349543));
#32922=CARTESIAN_POINT('Ctrl Pts',(19.3512124829545,-3.63381458932239,4.99340047650924));
#32923=CARTESIAN_POINT('Ctrl Pts',(18.9870650305019,-3.31269812051263,4.26678755349543));
#32924=CARTESIAN_POINT('Ctrl Pts',(19.6887012979566,-3.50544371457661,4.26678755349543));
#32925=CARTESIAN_POINT('Ctrl Pts',(19.4388776981255,-3.43572640272002,4.94574244817469));
#32926=CARTESIAN_POINT('Ctrl Pts',(19.0065895537831,-3.23231765789036,4.26678755349543));
#32927=CARTESIAN_POINT('Ctrl Pts',(19.6785000210075,-3.38383421296915,4.26678755349542));
#32928=CARTESIAN_POINT('Ctrl Pts',(19.4717925115843,-3.3358624643861,4.92141882649626));
#32929=CARTESIAN_POINT('Ctrl Pts',(19.0358080846578,-3.06916458966381,4.26678755349543));
#32930=CARTESIAN_POINT('Ctrl Pts',(19.6493709517514,-3.15527991967624,4.26678755349543));
#32931=CARTESIAN_POINT('Ctrl Pts',(19.5210828374545,-3.1358245681776,4.8721994557354));
#32932=CARTESIAN_POINT('Ctrl Pts',(19.0454759169275,-2.98595579110855,4.26678755349543));
#32933=CARTESIAN_POINT('Ctrl Pts',(19.6306860078638,-3.04632498898756,4.26678755349543));
#32934=CARTESIAN_POINT('Ctrl Pts',(19.5374124319044,-3.03513513584574,4.84717438865481));
#32935=CARTESIAN_POINT('Ctrl Pts',(19.0621241480217,-2.737285008801,4.26678755349543));
#32936=CARTESIAN_POINT('Ctrl Pts',(19.5687800824396,-2.74533278574744,4.26678755349543));
#32937=CARTESIAN_POINT('Ctrl Pts',(19.5656042620897,-2.7384688239187,4.77296272555879));
#32938=CARTESIAN_POINT('Ctrl Pts',(19.057271160227,-2.57250304610006,4.26678755349543));
#32939=CARTESIAN_POINT('Ctrl Pts',(19.5173428295347,-2.5555887020504,4.26678755349543));
#32940=CARTESIAN_POINT('Ctrl Pts',(19.5575361035113,-2.54753565754633,4.72455016526169));
#32941=CARTESIAN_POINT('Ctrl Pts',(19.0269269806048,-2.24423104073317,4.26678755349543));
#32942=CARTESIAN_POINT('Ctrl Pts',(19.4037324746258,-2.19827110756716,4.26678755349543));
#32943=CARTESIAN_POINT('Ctrl Pts',(19.5066380987991,-2.17857853420919,4.63172588697633));
#32944=CARTESIAN_POINT('Ctrl Pts',(19.0011662279257,-2.0804291629179,4.26678755349543));
#32945=CARTESIAN_POINT('Ctrl Pts',(19.3411771890505,-2.0261294786292,4.26678755349543));
#32946=CARTESIAN_POINT('Ctrl Pts',(19.463348919041,-2.0002486625875,4.58724452357084));
#32947=CARTESIAN_POINT('Ctrl Pts',(18.9022612159307,-1.59259935669663,4.26678755349543));
#32948=CARTESIAN_POINT('Ctrl Pts',(19.1484414382609,-1.54317772475002,4.26678755349543));
#32949=CARTESIAN_POINT('Ctrl Pts',(19.2970255960277,-1.48543183133247,4.46381231351943));
#32950=CARTESIAN_POINT('Ctrl Pts',(18.808053085376,-1.27510872906614,4.26678755349543));
#32951=CARTESIAN_POINT('Ctrl Pts',(18.9991637252048,-1.22485530444607,4.26678755349543));
#32952=CARTESIAN_POINT('Ctrl Pts',(19.1384956426123,-1.17248948697599,4.39571969599962));
#32953=CARTESIAN_POINT('Ctrl Pts',(18.65499946014,-0.802082822629942,4.26678755349543));
#32954=CARTESIAN_POINT('Ctrl Pts',(18.7752857128794,-0.764203897240211,
4.26678755349543));
#32955=CARTESIAN_POINT('Ctrl Pts',(18.8808742045249,-0.726828291197418,
4.32500544029631));
#32956=CARTESIAN_POINT('Ctrl Pts',(18.6014509972622,-0.645096921999107,
4.26678755349543));
#32957=CARTESIAN_POINT('Ctrl Pts',(18.7002177320532,-0.613472528045095,
4.26678755349542));
#32958=CARTESIAN_POINT('Ctrl Pts',(18.7907282330956,-0.582301152819928,
4.30665226666321));
#32959=CARTESIAN_POINT('Ctrl Pts',(18.5277457016062,-0.407818315284438,
4.26678755349543));
#32960=CARTESIAN_POINT('Ctrl Pts',(18.598737077538,-0.387068822042169,4.26678755349543));
#32961=CARTESIAN_POINT('Ctrl Pts',(18.6666415536194,-0.366671419750548,
4.28784256921206));
#32962=CARTESIAN_POINT('Ctrl Pts',(18.5042426057228,-0.328435858715446,
4.26678755349543));
#32963=CARTESIAN_POINT('Ctrl Pts',(18.5666903059424,-0.311580987664372,
4.26678755349543));
#32964=CARTESIAN_POINT('Ctrl Pts',(18.6270715338758,-0.294994221998134,
4.28301860951388));
#32965=CARTESIAN_POINT('Ctrl Pts',(18.4373471175324,-0.0378434116184329,
4.26678755349543));
#32966=CARTESIAN_POINT('Ctrl Pts',(18.4761993712803,-0.0366262354591573,
4.26678755349543));
#32967=CARTESIAN_POINT('Ctrl Pts',(18.5144427309313,-0.0335231859295633,
4.27116249911528));
#32968=CARTESIAN_POINT('Ctrl Pts',(18.4253014419183,0.186125192633141,4.26678755349543));
#32969=CARTESIAN_POINT('Ctrl Pts',(18.4597225256734,0.17753430427652,4.26678755349789));
#32970=CARTESIAN_POINT('Ctrl Pts',(18.4941622956095,0.166269977993189,4.2728958886403));
#32971=CARTESIAN_POINT('Ctrl Pts',(18.5875304087241,0.411880125146817,4.26678755349542));
#32972=CARTESIAN_POINT('Ctrl Pts',(18.6805827233783,0.39133576211092,4.26678755348346));
#32973=CARTESIAN_POINT('Ctrl Pts',(18.7672955102272,0.370166055980356,4.28926970183153));
#38614=UNCERTAINTY_MEASURE_WITH_UNIT(LENGTH_MEASURE(0.01),#38636,
'DISTANCE_ACCURACY_VALUE',
'Maximum model space distance between geometric entities at asserted c
onnectivities');
#38619=UNCERTAINTY_MEASURE_WITH_UNIT(LENGTH_MEASURE(0.01),#38636,
'DISTANCE_ACCURACY_VALUE',
'Maximum model space distance between geometric entities at asserted c
onnectivities');
#38630=(
GEOMETRIC_REPRESENTATION_CONTEXT(3)
GLOBAL_UNCERTAINTY_ASSIGNED_CONTEXT((#38614))
GLOBAL_UNIT_ASSIGNED_CONTEXT((#38636,#38638,#38639))
REPRESENTATION_CONTEXT('','3D')
);
#38635=(
GEOMETRIC_REPRESENTATION_CONTEXT(3)
GLOBAL_UNCERTAINTY_ASSIGNED_CONTEXT((#38619))
GLOBAL_UNIT_ASSIGNED_CONTEXT((#38636,#38638,#38639))
REPRESENTATION_CONTEXT('','3D')
);
#38636=(
LENGTH_UNIT()
NAMED_UNIT(*)
SI_UNIT(.MILLI.,.METRE.)
);
#38638=(
NAMED_UNIT(*)
PLANE_ANGLE_UNIT()
SI_UNIT($,.RADIAN.)
);
#38639=(
NAMED_UNIT(*)
SI_UNIT($,.STERADIAN.)
SOLID_ANGLE_UNIT()
);
#38650=SHAPE_DEFINITION_REPRESENTATION(#38665,#38694);
#38665=PRODUCT_DEFINITION_SHAPE('',$,#38710);
#38694=SHAPE_REPRESENTATION('',(#18149),#38630);
#38699=PRODUCT_DEFINITION_CONTEXT('part definition',#38746,'design');
#38710=PRODUCT_DEFINITION('Arm Joint 2','Arm Joint 2',#38725,#38699);
#38725=PRODUCT_DEFINITION_FORMATION('',$,#38758);
#38746=APPLICATION_CONTEXT(
'Core Data for Automotive Mechanical Design Process');
#38747=PRODUCT_CONTEXT('part definition',#38746,'mechanical');
#38758=PRODUCT('Arm Joint 2','Arm Joint 2',$,(#38747));
#38767=PRESENTATION_STYLE_ASSIGNMENT((#38774));
#38774=SURFACE_STYLE_USAGE(.BOTH.,#38781);
#38781=SURFACE_SIDE_STYLE('',(#38788));
#38788=SURFACE_STYLE_FILL_AREA(#38795);
#38795=FILL_AREA_STYLE('Opaque(97,158,199)',(#38802));
#38802=FILL_AREA_STYLE_COLOUR('Opaque(97,158,199)',#38809);
#38809=COLOUR_RGB('Opaque(97,158,199)',0.380392156862745,0.619607843137255,
0.780392156862745);
ENDSEC;
END-ISO-10303-21;
